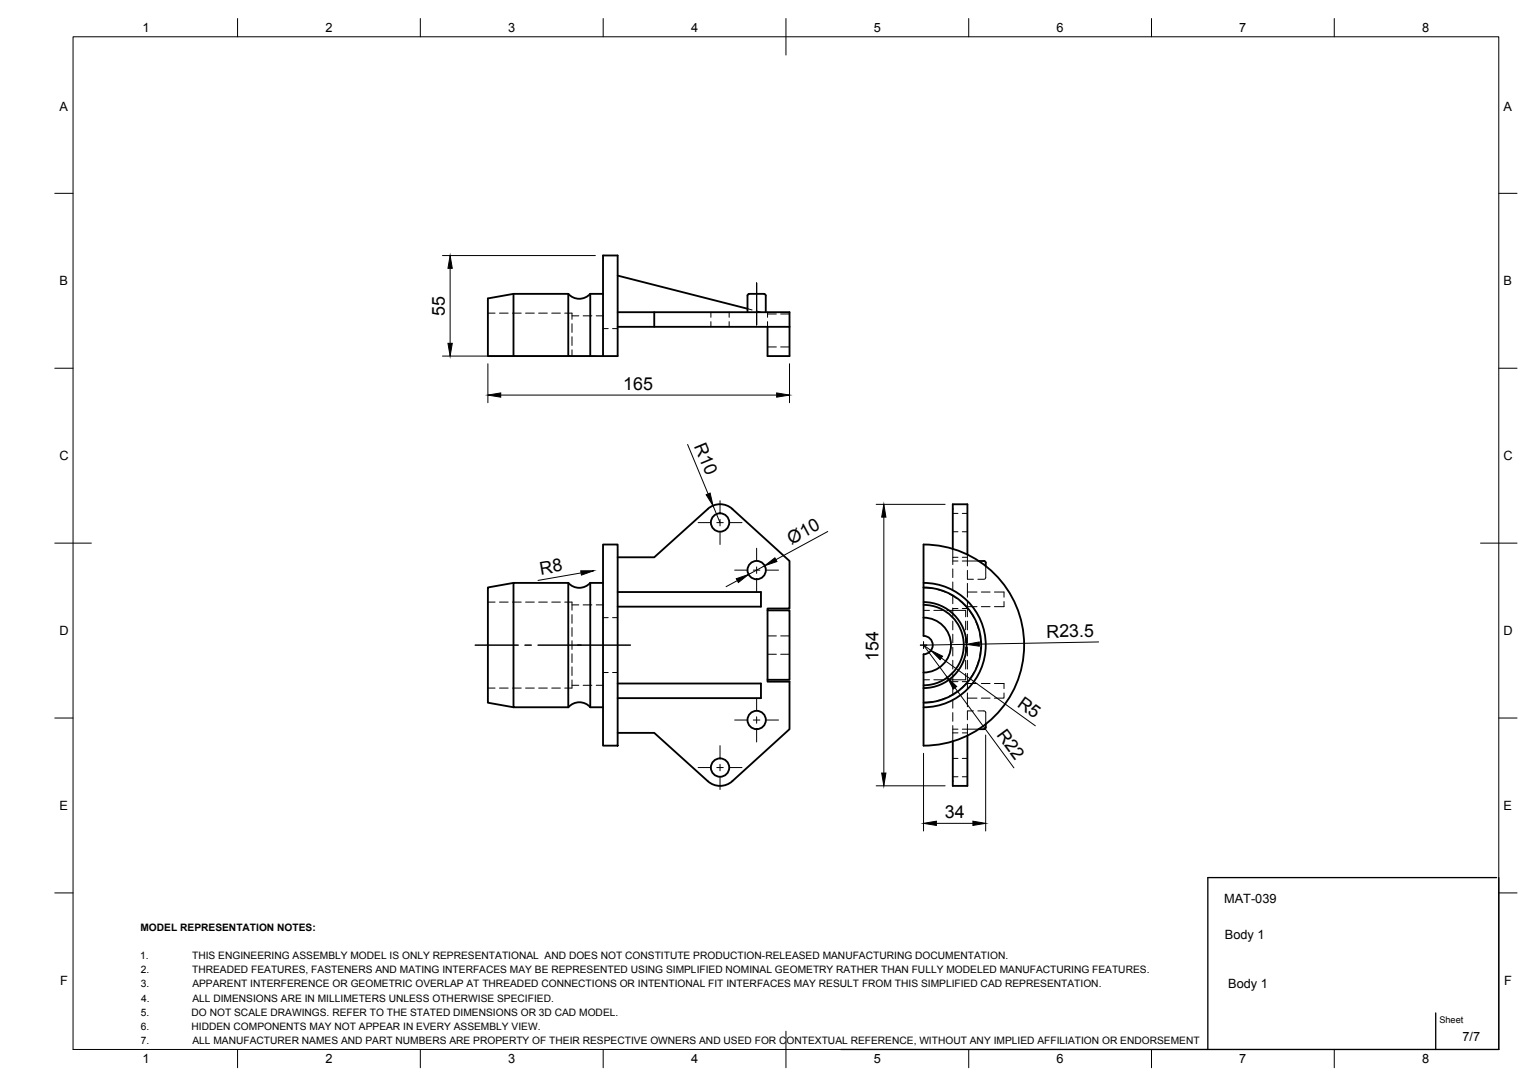
ISO-10303-21;
HEADER;
/* Generated by software containing ST-Developer
 * from STEP Tools, Inc. (www.steptools.com) 
 */

FILE_DESCRIPTION(
/* description */ ('STEP AP214'),
/* implementation_level */ '2;1');

FILE_NAME(
/* name */ 'Body 1.step',
/* time_stamp */ '2026-11-14T21:46:24-08:00',
/* author */ (''),
/* organization */ (''),
/* preprocessor_version */ 'ST-DEVELOPER v20.2',
/* originating_system */ 'Autodesk Translation Framework v15.17.0.0',
/* authorisation */ '');

FILE_SCHEMA (('AUTOMOTIVE_DESIGN { 1 0 10303 214 3 1 1 }'));
ENDSEC;

DATA;
#10=MECHANICAL_DESIGN_GEOMETRIC_PRESENTATION_REPRESENTATION('',(#89),#7783);
#75=SHAPE_REPRESENTATION_RELATIONSHIP('SRR','None',#7820,#82);
#82=ADVANCED_BREP_SHAPE_REPRESENTATION('',(#96),#7776);
#89=STYLED_ITEM('',(#7868),#96);
#96=MANIFOLD_SOLID_BREP('Body1',#4164);
#103=CONICAL_SURFACE('',#4303,34.,0.176708856070037);
#112=FACE_BOUND('',#1344,.T.);
#113=FACE_BOUND('',#1345,.T.);
#114=FACE_BOUND('',#1346,.T.);
#115=FACE_BOUND('',#1347,.T.);
#116=FACE_BOUND('',#1352,.T.);
#117=FACE_BOUND('',#1359,.T.);
#118=FACE_BOUND('',#1360,.T.);
#159=PLANE('',#4294);
#160=PLANE('',#4297);
#161=PLANE('',#4298);
#162=PLANE('',#4299);
#163=PLANE('',#4300);
#164=PLANE('',#4301);
#165=PLANE('',#4304);
#166=PLANE('',#4305);
#167=PLANE('',#4306);
#168=PLANE('',#4307);
#169=PLANE('',#4310);
#170=PLANE('',#4311);
#171=PLANE('',#4313);
#172=PLANE('',#4314);
#173=PLANE('',#4315);
#174=PLANE('',#4317);
#175=PLANE('',#4318);
#176=PLANE('',#4319);
#177=PLANE('',#4320);
#178=PLANE('',#4321);
#179=PLANE('',#4322);
#180=PLANE('',#4323);
#181=PLANE('',#4324);
#182=PLANE('',#4325);
#183=PLANE('',#4326);
#184=PLANE('',#4327);
#185=PLANE('',#4328);
#186=PLANE('',#4329);
#187=PLANE('',#4330);
#188=PLANE('',#4331);
#189=PLANE('',#4332);
#190=PLANE('',#4333);
#191=PLANE('',#4334);
#192=PLANE('',#4335);
#193=PLANE('',#4336);
#289=LINE('',#6018,#648);
#290=LINE('',#6028,#649);
#291=LINE('',#6034,#650);
#292=LINE('',#6037,#651);
#293=LINE('',#6042,#652);
#294=LINE('',#6048,#653);
#295=LINE('',#6055,#654);
#296=LINE('',#6058,#655);
#297=LINE('',#6064,#656);
#298=LINE('',#6067,#657);
#299=LINE('',#6073,#658);
#300=LINE('',#6076,#659);
#301=LINE('',#6082,#660);
#302=LINE('',#6085,#661);
#303=LINE('',#6090,#662);
#304=LINE('',#6091,#663);
#305=LINE('',#6094,#664);
#306=LINE('',#6097,#665);
#307=LINE('',#6101,#666);
#308=LINE('',#6103,#667);
#309=LINE('',#6105,#668);
#310=LINE('',#6107,#669);
#311=LINE('',#6109,#670);
#312=LINE('',#6113,#671);
#313=LINE('',#6115,#672);
#314=LINE('',#6117,#673);
#315=LINE('',#6119,#674);
#316=LINE('',#6121,#675);
#317=LINE('',#6123,#676);
#318=LINE('',#6125,#677);
#319=LINE('',#6127,#678);
#320=LINE('',#6129,#679);
#321=LINE('',#6131,#680);
#322=LINE('',#6133,#681);
#323=LINE('',#6135,#682);
#324=LINE('',#6137,#683);
#325=LINE('',#6141,#684);
#326=LINE('',#6142,#685);
#327=LINE('',#6145,#686);
#328=LINE('',#6146,#687);
#329=LINE('',#6147,#688);
#330=LINE('',#6148,#689);
#331=LINE('',#6149,#690);
#332=LINE('',#6150,#691);
#333=LINE('',#6154,#692);
#334=LINE('',#6156,#693);
#335=LINE('',#6158,#694);
#336=LINE('',#6160,#695);
#337=LINE('',#6162,#696);
#338=LINE('',#6163,#697);
#339=LINE('',#6164,#698);
#340=LINE('',#6168,#699);
#341=LINE('',#6169,#700);
#342=LINE('',#6170,#701);
#343=LINE('',#6172,#702);
#344=LINE('',#6174,#703);
#345=LINE('',#6176,#704);
#346=LINE('',#6177,#705);
#347=LINE('',#6179,#706);
#348=LINE('',#6181,#707);
#349=LINE('',#6182,#708);
#350=LINE('',#6184,#709);
#351=LINE('',#6186,#710);
#352=LINE('',#6187,#711);
#353=LINE('',#6191,#712);
#354=LINE('',#6193,#713);
#355=LINE('',#6195,#714);
#356=LINE('',#6197,#715);
#357=LINE('',#6199,#716);
#358=LINE('',#6201,#717);
#359=LINE('',#6203,#718);
#360=LINE('',#6207,#719);
#361=LINE('',#6208,#720);
#362=LINE('',#6210,#721);
#363=LINE('',#6212,#722);
#364=LINE('',#6216,#723);
#365=LINE('',#6218,#724);
#366=LINE('',#6219,#725);
#367=LINE('',#6220,#726);
#368=LINE('',#6222,#727);
#369=LINE('',#6224,#728);
#370=LINE('',#6226,#729);
#371=LINE('',#6229,#730);
#372=LINE('',#6230,#731);
#373=LINE('',#6232,#732);
#374=LINE('',#6234,#733);
#375=LINE('',#6236,#734);
#376=LINE('',#6239,#735);
#377=LINE('',#6240,#736);
#378=LINE('',#6244,#737);
#379=LINE('',#6245,#738);
#380=LINE('',#6252,#739);
#381=LINE('',#6253,#740);
#382=LINE('',#6255,#741);
#383=LINE('',#6256,#742);
#384=LINE('',#6259,#743);
#385=LINE('',#6261,#744);
#386=LINE('',#6263,#745);
#387=LINE('',#6265,#746);
#388=LINE('',#6266,#747);
#389=LINE('',#6268,#748);
#390=LINE('',#6269,#749);
#391=LINE('',#6271,#750);
#392=LINE('',#6273,#751);
#648=VECTOR('',#4740,5.00000000000003);
#649=VECTOR('',#4753,5.00000000000003);
#650=VECTOR('',#4758,1000.);
#651=VECTOR('',#4761,1000.);
#652=VECTOR('',#4766,5.00000000000002);
#653=VECTOR('',#4773,5.00000000000002);
#654=VECTOR('',#4780,1000.);
#655=VECTOR('',#4783,1000.);
#656=VECTOR('',#4788,1000.);
#657=VECTOR('',#4791,1000.);
#658=VECTOR('',#4796,1000.);
#659=VECTOR('',#4799,1000.);
#660=VECTOR('',#4804,1000.);
#661=VECTOR('',#4807,1000.);
#662=VECTOR('',#4812,1000.);
#663=VECTOR('',#4813,1000.);
#664=VECTOR('',#4816,1000.);
#665=VECTOR('',#4819,1000.);
#666=VECTOR('',#4822,1000.);
#667=VECTOR('',#4823,1000.);
#668=VECTOR('',#4824,1000.);
#669=VECTOR('',#4825,1000.);
#670=VECTOR('',#4826,1000.);
#671=VECTOR('',#4829,1000.);
#672=VECTOR('',#4830,1000.);
#673=VECTOR('',#4831,1000.);
#674=VECTOR('',#4832,1000.);
#675=VECTOR('',#4833,1000.);
#676=VECTOR('',#4834,1000.);
#677=VECTOR('',#4835,1000.);
#678=VECTOR('',#4836,1000.);
#679=VECTOR('',#4837,1000.);
#680=VECTOR('',#4838,1000.);
#681=VECTOR('',#4839,1000.);
#682=VECTOR('',#4840,1000.);
#683=VECTOR('',#4841,1000.);
#684=VECTOR('',#4844,1000.);
#685=VECTOR('',#4845,1000.);
#686=VECTOR('',#4848,1000.);
#687=VECTOR('',#4849,1000.);
#688=VECTOR('',#4850,1000.);
#689=VECTOR('',#4851,1000.);
#690=VECTOR('',#4852,1000.);
#691=VECTOR('',#4853,1000.);
#692=VECTOR('',#4856,1000.);
#693=VECTOR('',#4857,1000.);
#694=VECTOR('',#4858,1000.);
#695=VECTOR('',#4859,1000.);
#696=VECTOR('',#4860,1000.);
#697=VECTOR('',#4861,1000.);
#698=VECTOR('',#4862,1000.);
#699=VECTOR('',#4865,1000.);
#700=VECTOR('',#4866,1000.);
#701=VECTOR('',#4867,1000.);
#702=VECTOR('',#4870,1000.);
#703=VECTOR('',#4871,1000.);
#704=VECTOR('',#4872,1000.);
#705=VECTOR('',#4873,1000.);
#706=VECTOR('',#4874,1000.);
#707=VECTOR('',#4875,1000.);
#708=VECTOR('',#4876,1000.);
#709=VECTOR('',#4877,1000.);
#710=VECTOR('',#4878,1000.);
#711=VECTOR('',#4879,1000.);
#712=VECTOR('',#4884,1000.);
#713=VECTOR('',#4887,1000.);
#714=VECTOR('',#4890,1000.);
#715=VECTOR('',#4893,1000.);
#716=VECTOR('',#4896,1000.);
#717=VECTOR('',#4899,1000.);
#718=VECTOR('',#4900,1000.);
#719=VECTOR('',#4903,1000.);
#720=VECTOR('',#4904,1000.);
#721=VECTOR('',#4905,1000.);
#722=VECTOR('',#4906,1000.);
#723=VECTOR('',#4909,1000.);
#724=VECTOR('',#4910,1000.);
#725=VECTOR('',#4911,1000.);
#726=VECTOR('',#4912,1000.);
#727=VECTOR('',#4915,1000.);
#728=VECTOR('',#4918,1000.);
#729=VECTOR('',#4921,1000.);
#730=VECTOR('',#4926,1000.);
#731=VECTOR('',#4927,1000.);
#732=VECTOR('',#4930,1000.);
#733=VECTOR('',#4933,1000.);
#734=VECTOR('',#4936,1000.);
#735=VECTOR('',#4941,1000.);
#736=VECTOR('',#4942,1000.);
#737=VECTOR('',#4949,1000.);
#738=VECTOR('',#4950,1000.);
#739=VECTOR('',#4961,1000.);
#740=VECTOR('',#4962,1000.);
#741=VECTOR('',#4963,1000.);
#742=VECTOR('',#4964,1000.);
#743=VECTOR('',#4967,1000.);
#744=VECTOR('',#4968,1000.);
#745=VECTOR('',#4969,1000.);
#746=VECTOR('',#4970,1000.);
#747=VECTOR('',#4971,1000.);
#748=VECTOR('',#4974,1000.);
#749=VECTOR('',#4975,1000.);
#750=VECTOR('',#4978,1000.);
#751=VECTOR('',#4981,1000.);
#1007=CYLINDRICAL_SURFACE('',#4261,5.00000000000003);
#1008=CYLINDRICAL_SURFACE('',#4267,5.00000000000003);
#1009=CYLINDRICAL_SURFACE('',#4269,5.);
#1010=CYLINDRICAL_SURFACE('',#4272,5.00000000000002);
#1011=CYLINDRICAL_SURFACE('',#4275,5.00000000000002);
#1012=CYLINDRICAL_SURFACE('',#4278,23.5);
#1013=CYLINDRICAL_SURFACE('',#4281,22.);
#1014=CYLINDRICAL_SURFACE('',#4284,15.);
#1015=CYLINDRICAL_SURFACE('',#4287,55.);
#1016=CYLINDRICAL_SURFACE('',#4290,34.);
#1017=CYLINDRICAL_SURFACE('',#4292,34.);
#1018=CYLINDRICAL_SURFACE('',#4312,10.);
#1019=CYLINDRICAL_SURFACE('',#4316,10.);
#1086=FACE_OUTER_BOUND('',#1329,.T.);
#1087=FACE_OUTER_BOUND('',#1330,.T.);
#1088=FACE_OUTER_BOUND('',#1331,.T.);
#1089=FACE_OUTER_BOUND('',#1332,.T.);
#1090=FACE_OUTER_BOUND('',#1333,.T.);
#1091=FACE_OUTER_BOUND('',#1334,.T.);
#1092=FACE_OUTER_BOUND('',#1335,.T.);
#1093=FACE_OUTER_BOUND('',#1336,.T.);
#1094=FACE_OUTER_BOUND('',#1337,.T.);
#1095=FACE_OUTER_BOUND('',#1338,.T.);
#1096=FACE_OUTER_BOUND('',#1339,.T.);
#1097=FACE_OUTER_BOUND('',#1340,.T.);
#1098=FACE_OUTER_BOUND('',#1341,.T.);
#1099=FACE_OUTER_BOUND('',#1342,.T.);
#1100=FACE_OUTER_BOUND('',#1343,.T.);
#1101=FACE_OUTER_BOUND('',#1348,.T.);
#1102=FACE_OUTER_BOUND('',#1349,.T.);
#1103=FACE_OUTER_BOUND('',#1350,.T.);
#1104=FACE_OUTER_BOUND('',#1351,.T.);
#1105=FACE_OUTER_BOUND('',#1353,.T.);
#1106=FACE_OUTER_BOUND('',#1354,.T.);
#1107=FACE_OUTER_BOUND('',#1355,.T.);
#1108=FACE_OUTER_BOUND('',#1356,.T.);
#1109=FACE_OUTER_BOUND('',#1357,.T.);
#1110=FACE_OUTER_BOUND('',#1358,.T.);
#1111=FACE_OUTER_BOUND('',#1361,.T.);
#1112=FACE_OUTER_BOUND('',#1362,.T.);
#1113=FACE_OUTER_BOUND('',#1363,.T.);
#1114=FACE_OUTER_BOUND('',#1364,.T.);
#1115=FACE_OUTER_BOUND('',#1365,.T.);
#1116=FACE_OUTER_BOUND('',#1366,.T.);
#1117=FACE_OUTER_BOUND('',#1367,.T.);
#1118=FACE_OUTER_BOUND('',#1368,.T.);
#1119=FACE_OUTER_BOUND('',#1369,.T.);
#1120=FACE_OUTER_BOUND('',#1370,.T.);
#1121=FACE_OUTER_BOUND('',#1371,.T.);
#1122=FACE_OUTER_BOUND('',#1372,.T.);
#1123=FACE_OUTER_BOUND('',#1373,.T.);
#1124=FACE_OUTER_BOUND('',#1374,.T.);
#1125=FACE_OUTER_BOUND('',#1375,.T.);
#1126=FACE_OUTER_BOUND('',#1376,.T.);
#1127=FACE_OUTER_BOUND('',#1377,.T.);
#1128=FACE_OUTER_BOUND('',#1378,.T.);
#1129=FACE_OUTER_BOUND('',#1379,.T.);
#1130=FACE_OUTER_BOUND('',#1380,.T.);
#1131=FACE_OUTER_BOUND('',#1381,.T.);
#1132=FACE_OUTER_BOUND('',#1382,.T.);
#1133=FACE_OUTER_BOUND('',#1383,.T.);
#1134=FACE_OUTER_BOUND('',#1384,.T.);
#1135=FACE_OUTER_BOUND('',#1385,.T.);
#1136=FACE_OUTER_BOUND('',#1386,.T.);
#1137=FACE_OUTER_BOUND('',#1387,.T.);
#1329=EDGE_LOOP('',(#2758,#2759,#2760,#2761));
#1330=EDGE_LOOP('',(#2762,#2763,#2764,#2765));
#1331=EDGE_LOOP('',(#2766,#2767,#2768,#2769));
#1332=EDGE_LOOP('',(#2770,#2771,#2772,#2773));
#1333=EDGE_LOOP('',(#2774,#2775,#2776,#2777));
#1334=EDGE_LOOP('',(#2778,#2779,#2780,#2781));
#1335=EDGE_LOOP('',(#2782,#2783,#2784,#2785));
#1336=EDGE_LOOP('',(#2786,#2787,#2788,#2789));
#1337=EDGE_LOOP('',(#2790,#2791,#2792,#2793));
#1338=EDGE_LOOP('',(#2794,#2795,#2796,#2797));
#1339=EDGE_LOOP('',(#2798,#2799,#2800,#2801));
#1340=EDGE_LOOP('',(#2802,#2803,#2804,#2805));
#1341=EDGE_LOOP('',(#2806,#2807,#2808,#2809));
#1342=EDGE_LOOP('',(#2810,#2811,#2812,#2813));
#1343=EDGE_LOOP('',(#2814,#2815,#2816,#2817,#2818,#2819,#2820,#2821,#2822,
#2823,#2824,#2825,#2826,#2827,#2828,#2829,#2830,#2831,#2832,#2833,#2834,
#2835));
#1344=EDGE_LOOP('',(#2836));
#1345=EDGE_LOOP('',(#2837));
#1346=EDGE_LOOP('',(#2838));
#1347=EDGE_LOOP('',(#2839));
#1348=EDGE_LOOP('',(#2840,#2841,#2842,#2843,#2844,#2845,#2846,#2847,#2848,
#2849,#2850,#2851,#2852));
#1349=EDGE_LOOP('',(#2853,#2854,#2855,#2856,#2857,#2858,#2859,#2860));
#1350=EDGE_LOOP('',(#2861,#2862,#2863,#2864));
#1351=EDGE_LOOP('',(#2865,#2866,#2867,#2868));
#1352=EDGE_LOOP('',(#2869,#2870,#2871,#2872,#2873,#2874,#2875,#2876,#2877,
#2878,#2879,#2880));
#1353=EDGE_LOOP('',(#2881,#2882,#2883,#2884));
#1354=EDGE_LOOP('',(#2885,#2886,#2887,#2888));
#1355=EDGE_LOOP('',(#2889,#2890,#2891,#2892));
#1356=EDGE_LOOP('',(#2893,#2894,#2895,#2896));
#1357=EDGE_LOOP('',(#2897,#2898,#2899,#2900));
#1358=EDGE_LOOP('',(#2901,#2902,#2903,#2904,#2905,#2906,#2907,#2908,#2909,
#2910,#2911,#2912,#2913,#2914,#2915,#2916));
#1359=EDGE_LOOP('',(#2917));
#1360=EDGE_LOOP('',(#2918));
#1361=EDGE_LOOP('',(#2919,#2920,#2921,#2922));
#1362=EDGE_LOOP('',(#2923,#2924,#2925,#2926));
#1363=EDGE_LOOP('',(#2927,#2928,#2929,#2930));
#1364=EDGE_LOOP('',(#2931,#2932,#2933,#2934));
#1365=EDGE_LOOP('',(#2935,#2936,#2937,#2938));
#1366=EDGE_LOOP('',(#2939,#2940,#2941,#2942));
#1367=EDGE_LOOP('',(#2943,#2944,#2945,#2946));
#1368=EDGE_LOOP('',(#2947,#2948,#2949,#2950));
#1369=EDGE_LOOP('',(#2951,#2952,#2953,#2954));
#1370=EDGE_LOOP('',(#2955,#2956,#2957,#2958));
#1371=EDGE_LOOP('',(#2959,#2960,#2961));
#1372=EDGE_LOOP('',(#2962,#2963,#2964));
#1373=EDGE_LOOP('',(#2965,#2966,#2967,#2968));
#1374=EDGE_LOOP('',(#2969,#2970,#2971));
#1375=EDGE_LOOP('',(#2972,#2973,#2974));
#1376=EDGE_LOOP('',(#2975,#2976,#2977,#2978));
#1377=EDGE_LOOP('',(#2979,#2980,#2981,#2982));
#1378=EDGE_LOOP('',(#2983,#2984,#2985,#2986,#2987,#2988));
#1379=EDGE_LOOP('',(#2989,#2990,#2991,#2992,#2993,#2994));
#1380=EDGE_LOOP('',(#2995,#2996,#2997,#2998));
#1381=EDGE_LOOP('',(#2999,#3000,#3001,#3002,#3003));
#1382=EDGE_LOOP('',(#3004,#3005,#3006,#3007,#3008));
#1383=EDGE_LOOP('',(#3009,#3010,#3011,#3012));
#1384=EDGE_LOOP('',(#3013,#3014,#3015,#3016,#3017,#3018,#3019,#3020,#3021,
#3022,#3023,#3024,#3025));
#1385=EDGE_LOOP('',(#3026,#3027,#3028,#3029));
#1386=EDGE_LOOP('',(#3030));
#1387=EDGE_LOOP('',(#3031));
#1619=CIRCLE('',#4253,8.);
#1620=CIRCLE('',#4254,34.);
#1621=CIRCLE('',#4255,8.);
#1622=CIRCLE('',#4256,34.);
#1623=CIRCLE('',#4258,5.00000000000003);
#1624=CIRCLE('',#4259,1.);
#1625=CIRCLE('',#4260,4.00000000000003);
#1626=CIRCLE('',#4262,5.00000000000003);
#1627=CIRCLE('',#4264,5.00000000000003);
#1628=CIRCLE('',#4265,1.);
#1629=CIRCLE('',#4266,4.00000000000003);
#1630=CIRCLE('',#4268,5.00000000000003);
#1631=CIRCLE('',#4270,5.);
#1632=CIRCLE('',#4271,5.);
#1633=CIRCLE('',#4273,5.00000000000002);
#1634=CIRCLE('',#4274,5.00000000000002);
#1635=CIRCLE('',#4276,5.00000000000003);
#1636=CIRCLE('',#4277,5.00000000000003);
#1637=CIRCLE('',#4279,23.5);
#1638=CIRCLE('',#4280,23.5);
#1639=CIRCLE('',#4282,22.);
#1640=CIRCLE('',#4283,22.);
#1641=CIRCLE('',#4285,15.);
#1642=CIRCLE('',#4286,15.);
#1643=CIRCLE('',#4288,55.);
#1644=CIRCLE('',#4289,55.);
#1645=CIRCLE('',#4291,34.);
#1646=CIRCLE('',#4293,34.);
#1647=CIRCLE('',#4295,10.);
#1648=CIRCLE('',#4296,10.);
#1649=CIRCLE('',#4302,31.5);
#1650=CIRCLE('',#4308,10.);
#1651=CIRCLE('',#4309,10.);
#1822=VERTEX_POINT('',#6001);
#1823=VERTEX_POINT('',#6002);
#1824=VERTEX_POINT('',#6004);
#1825=VERTEX_POINT('',#6006);
#1826=VERTEX_POINT('',#6010);
#1827=VERTEX_POINT('',#6012);
#1828=VERTEX_POINT('',#6016);
#1829=VERTEX_POINT('',#6020);
#1830=VERTEX_POINT('',#6022);
#1831=VERTEX_POINT('',#6026);
#1832=VERTEX_POINT('',#6030);
#1833=VERTEX_POINT('',#6031);
#1834=VERTEX_POINT('',#6033);
#1835=VERTEX_POINT('',#6035);
#1836=VERTEX_POINT('',#6039);
#1837=VERTEX_POINT('',#6041);
#1838=VERTEX_POINT('',#6045);
#1839=VERTEX_POINT('',#6047);
#1840=VERTEX_POINT('',#6051);
#1841=VERTEX_POINT('',#6052);
#1842=VERTEX_POINT('',#6054);
#1843=VERTEX_POINT('',#6056);
#1844=VERTEX_POINT('',#6060);
#1845=VERTEX_POINT('',#6061);
#1846=VERTEX_POINT('',#6063);
#1847=VERTEX_POINT('',#6065);
#1848=VERTEX_POINT('',#6069);
#1849=VERTEX_POINT('',#6070);
#1850=VERTEX_POINT('',#6072);
#1851=VERTEX_POINT('',#6074);
#1852=VERTEX_POINT('',#6078);
#1853=VERTEX_POINT('',#6079);
#1854=VERTEX_POINT('',#6081);
#1855=VERTEX_POINT('',#6083);
#1856=VERTEX_POINT('',#6087);
#1857=VERTEX_POINT('',#6088);
#1858=VERTEX_POINT('',#6093);
#1859=VERTEX_POINT('',#6095);
#1860=VERTEX_POINT('',#6099);
#1861=VERTEX_POINT('',#6100);
#1862=VERTEX_POINT('',#6102);
#1863=VERTEX_POINT('',#6104);
#1864=VERTEX_POINT('',#6106);
#1865=VERTEX_POINT('',#6108);
#1866=VERTEX_POINT('',#6110);
#1867=VERTEX_POINT('',#6112);
#1868=VERTEX_POINT('',#6114);
#1869=VERTEX_POINT('',#6116);
#1870=VERTEX_POINT('',#6118);
#1871=VERTEX_POINT('',#6120);
#1872=VERTEX_POINT('',#6122);
#1873=VERTEX_POINT('',#6124);
#1874=VERTEX_POINT('',#6126);
#1875=VERTEX_POINT('',#6128);
#1876=VERTEX_POINT('',#6130);
#1877=VERTEX_POINT('',#6132);
#1878=VERTEX_POINT('',#6134);
#1879=VERTEX_POINT('',#6136);
#1880=VERTEX_POINT('',#6138);
#1881=VERTEX_POINT('',#6140);
#1882=VERTEX_POINT('',#6144);
#1883=VERTEX_POINT('',#6152);
#1884=VERTEX_POINT('',#6153);
#1885=VERTEX_POINT('',#6155);
#1886=VERTEX_POINT('',#6157);
#1887=VERTEX_POINT('',#6159);
#1888=VERTEX_POINT('',#6161);
#1889=VERTEX_POINT('',#6166);
#1890=VERTEX_POINT('',#6167);
#1891=VERTEX_POINT('',#6173);
#1892=VERTEX_POINT('',#6175);
#1893=VERTEX_POINT('',#6178);
#1894=VERTEX_POINT('',#6180);
#1895=VERTEX_POINT('',#6183);
#1896=VERTEX_POINT('',#6185);
#1897=VERTEX_POINT('',#6189);
#1898=VERTEX_POINT('',#6202);
#1899=VERTEX_POINT('',#6204);
#1900=VERTEX_POINT('',#6206);
#1901=VERTEX_POINT('',#6209);
#1902=VERTEX_POINT('',#6211);
#1903=VERTEX_POINT('',#6213);
#1904=VERTEX_POINT('',#6215);
#1905=VERTEX_POINT('',#6217);
#1906=VERTEX_POINT('',#6251);
#1907=VERTEX_POINT('',#6254);
#1908=VERTEX_POINT('',#6258);
#1909=VERTEX_POINT('',#6260);
#1910=VERTEX_POINT('',#6262);
#1911=VERTEX_POINT('',#6264);
#2186=EDGE_CURVE('',#1822,#1823,#1619,.T.);
#2187=EDGE_CURVE('',#1823,#1824,#1620,.T.);
#2188=EDGE_CURVE('',#1824,#1825,#1621,.T.);
#2189=EDGE_CURVE('',#1822,#1825,#1622,.T.);
#2190=EDGE_CURVE('',#1826,#1826,#1623,.T.);
#2191=EDGE_CURVE('',#1826,#1827,#1624,.T.);
#2192=EDGE_CURVE('',#1827,#1827,#1625,.T.);
#2193=EDGE_CURVE('',#1828,#1828,#1626,.T.);
#2194=EDGE_CURVE('',#1828,#1826,#289,.T.);
#2195=EDGE_CURVE('',#1829,#1829,#1627,.T.);
#2196=EDGE_CURVE('',#1829,#1830,#1628,.T.);
#2197=EDGE_CURVE('',#1830,#1830,#1629,.T.);
#2198=EDGE_CURVE('',#1831,#1831,#1630,.T.);
#2199=EDGE_CURVE('',#1831,#1829,#290,.T.);
#2200=EDGE_CURVE('',#1832,#1833,#1631,.T.);
#2201=EDGE_CURVE('',#1834,#1833,#291,.T.);
#2202=EDGE_CURVE('',#1835,#1834,#1632,.T.);
#2203=EDGE_CURVE('',#1832,#1835,#292,.T.);
#2204=EDGE_CURVE('',#1836,#1836,#1633,.T.);
#2205=EDGE_CURVE('',#1836,#1837,#293,.T.);
#2206=EDGE_CURVE('',#1837,#1837,#1634,.T.);
#2207=EDGE_CURVE('',#1838,#1838,#1635,.T.);
#2208=EDGE_CURVE('',#1838,#1839,#294,.T.);
#2209=EDGE_CURVE('',#1839,#1839,#1636,.T.);
#2210=EDGE_CURVE('',#1840,#1841,#1637,.T.);
#2211=EDGE_CURVE('',#1840,#1842,#295,.T.);
#2212=EDGE_CURVE('',#1842,#1843,#1638,.T.);
#2213=EDGE_CURVE('',#1843,#1841,#296,.T.);
#2214=EDGE_CURVE('',#1844,#1845,#1639,.T.);
#2215=EDGE_CURVE('',#1844,#1846,#297,.T.);
#2216=EDGE_CURVE('',#1846,#1847,#1640,.T.);
#2217=EDGE_CURVE('',#1847,#1845,#298,.T.);
#2218=EDGE_CURVE('',#1848,#1849,#1641,.T.);
#2219=EDGE_CURVE('',#1848,#1850,#299,.T.);
#2220=EDGE_CURVE('',#1850,#1851,#1642,.T.);
#2221=EDGE_CURVE('',#1851,#1849,#300,.T.);
#2222=EDGE_CURVE('',#1852,#1853,#1643,.T.);
#2223=EDGE_CURVE('',#1853,#1854,#301,.T.);
#2224=EDGE_CURVE('',#1855,#1854,#1644,.T.);
#2225=EDGE_CURVE('',#1855,#1852,#302,.T.);
#2226=EDGE_CURVE('',#1856,#1857,#1645,.T.);
#2227=EDGE_CURVE('',#1857,#1824,#303,.T.);
#2228=EDGE_CURVE('',#1823,#1856,#304,.T.);
#2229=EDGE_CURVE('',#1825,#1858,#305,.T.);
#2230=EDGE_CURVE('',#1859,#1858,#1646,.T.);
#2231=EDGE_CURVE('',#1859,#1822,#306,.T.);
#2232=EDGE_CURVE('',#1860,#1861,#307,.T.);
#2233=EDGE_CURVE('',#1862,#1860,#308,.T.);
#2234=EDGE_CURVE('',#1862,#1863,#309,.T.);
#2235=EDGE_CURVE('',#1863,#1864,#310,.T.);
#2236=EDGE_CURVE('',#1864,#1865,#311,.T.);
#2237=EDGE_CURVE('',#1865,#1866,#1647,.T.);
#2238=EDGE_CURVE('',#1866,#1867,#312,.T.);
#2239=EDGE_CURVE('',#1867,#1868,#313,.T.);
#2240=EDGE_CURVE('',#1868,#1869,#314,.T.);
#2241=EDGE_CURVE('',#1870,#1869,#315,.T.);
#2242=EDGE_CURVE('',#1870,#1871,#316,.T.);
#2243=EDGE_CURVE('',#1871,#1872,#317,.T.);
#2244=EDGE_CURVE('',#1872,#1873,#318,.T.);
#2245=EDGE_CURVE('',#1874,#1873,#319,.T.);
#2246=EDGE_CURVE('',#1875,#1874,#320,.T.);
#2247=EDGE_CURVE('',#1875,#1876,#321,.T.);
#2248=EDGE_CURVE('',#1876,#1877,#322,.T.);
#2249=EDGE_CURVE('',#1877,#1878,#323,.T.);
#2250=EDGE_CURVE('',#1878,#1879,#324,.T.);
#2251=EDGE_CURVE('',#1879,#1880,#1648,.T.);
#2252=EDGE_CURVE('',#1880,#1881,#325,.T.);
#2253=EDGE_CURVE('',#1881,#1861,#326,.T.);
#2254=EDGE_CURVE('',#1858,#1882,#327,.T.);
#2255=EDGE_CURVE('',#1854,#1857,#328,.T.);
#2256=EDGE_CURVE('',#1849,#1853,#329,.T.);
#2257=EDGE_CURVE('',#1845,#1851,#330,.T.);
#2258=EDGE_CURVE('',#1841,#1847,#331,.T.);
#2259=EDGE_CURVE('',#1882,#1843,#332,.T.);
#2260=EDGE_CURVE('',#1883,#1884,#333,.T.);
#2261=EDGE_CURVE('',#1885,#1884,#334,.T.);
#2262=EDGE_CURVE('',#1886,#1885,#335,.T.);
#2263=EDGE_CURVE('',#1886,#1887,#336,.T.);
#2264=EDGE_CURVE('',#1887,#1888,#337,.T.);
#2265=EDGE_CURVE('',#1888,#1862,#338,.T.);
#2266=EDGE_CURVE('',#1860,#1883,#339,.T.);
#2267=EDGE_CURVE('',#1889,#1890,#340,.T.);
#2268=EDGE_CURVE('',#1861,#1890,#341,.T.);
#2269=EDGE_CURVE('',#1881,#1889,#342,.T.);
#2270=EDGE_CURVE('',#1852,#1848,#343,.T.);
#2271=EDGE_CURVE('',#1876,#1891,#344,.T.);
#2272=EDGE_CURVE('',#1891,#1892,#345,.T.);
#2273=EDGE_CURVE('',#1873,#1892,#346,.T.);
#2274=EDGE_CURVE('',#1872,#1893,#347,.T.);
#2275=EDGE_CURVE('',#1894,#1893,#348,.T.);
#2276=EDGE_CURVE('',#1869,#1894,#349,.T.);
#2277=EDGE_CURVE('',#1868,#1895,#350,.T.);
#2278=EDGE_CURVE('',#1895,#1896,#351,.T.);
#2279=EDGE_CURVE('',#1877,#1896,#352,.T.);
#2280=EDGE_CURVE('',#1897,#1882,#1649,.T.);
#2281=EDGE_CURVE('',#1842,#1897,#353,.T.);
#2282=EDGE_CURVE('',#1897,#1859,#354,.T.);
#2283=EDGE_CURVE('',#1856,#1855,#355,.T.);
#2284=EDGE_CURVE('',#1850,#1844,#356,.T.);
#2285=EDGE_CURVE('',#1846,#1840,#357,.T.);
#2286=EDGE_CURVE('',#1883,#1890,#358,.T.);
#2287=EDGE_CURVE('',#1898,#1889,#359,.T.);
#2288=EDGE_CURVE('',#1899,#1898,#1650,.T.);
#2289=EDGE_CURVE('',#1900,#1899,#360,.T.);
#2290=EDGE_CURVE('',#1896,#1900,#361,.T.);
#2291=EDGE_CURVE('',#1901,#1895,#362,.T.);
#2292=EDGE_CURVE('',#1902,#1901,#363,.T.);
#2293=EDGE_CURVE('',#1903,#1902,#1651,.T.);
#2294=EDGE_CURVE('',#1904,#1903,#364,.T.);
#2295=EDGE_CURVE('',#1905,#1904,#365,.T.);
#2296=EDGE_CURVE('',#1905,#1888,#366,.T.);
#2297=EDGE_CURVE('',#1884,#1887,#367,.T.);
#2298=EDGE_CURVE('',#1878,#1900,#368,.T.);
#2299=EDGE_CURVE('',#1879,#1899,#369,.T.);
#2300=EDGE_CURVE('',#1880,#1898,#370,.T.);
#2301=EDGE_CURVE('',#1905,#1863,#371,.T.);
#2302=EDGE_CURVE('',#1864,#1904,#372,.T.);
#2303=EDGE_CURVE('',#1865,#1903,#373,.T.);
#2304=EDGE_CURVE('',#1866,#1902,#374,.T.);
#2305=EDGE_CURVE('',#1867,#1901,#375,.T.);
#2306=EDGE_CURVE('',#1893,#1871,#376,.T.);
#2307=EDGE_CURVE('',#1894,#1870,#377,.T.);
#2308=EDGE_CURVE('',#1892,#1874,#378,.T.);
#2309=EDGE_CURVE('',#1891,#1875,#379,.T.);
#2310=EDGE_CURVE('',#1906,#1887,#380,.T.);
#2311=EDGE_CURVE('',#1906,#1835,#381,.T.);
#2312=EDGE_CURVE('',#1834,#1907,#382,.T.);
#2313=EDGE_CURVE('',#1884,#1907,#383,.T.);
#2314=EDGE_CURVE('',#1908,#1832,#384,.T.);
#2315=EDGE_CURVE('',#1908,#1909,#385,.T.);
#2316=EDGE_CURVE('',#1909,#1910,#386,.T.);
#2317=EDGE_CURVE('',#1910,#1911,#387,.T.);
#2318=EDGE_CURVE('',#1833,#1911,#388,.T.);
#2319=EDGE_CURVE('',#1910,#1885,#389,.T.);
#2320=EDGE_CURVE('',#1909,#1886,#390,.T.);
#2321=EDGE_CURVE('',#1907,#1911,#391,.T.);
#2322=EDGE_CURVE('',#1908,#1906,#392,.T.);
#2758=ORIENTED_EDGE('',*,*,#2186,.T.);
#2759=ORIENTED_EDGE('',*,*,#2187,.T.);
#2760=ORIENTED_EDGE('',*,*,#2188,.T.);
#2761=ORIENTED_EDGE('',*,*,#2189,.F.);
#2762=ORIENTED_EDGE('',*,*,#2190,.F.);
#2763=ORIENTED_EDGE('',*,*,#2191,.T.);
#2764=ORIENTED_EDGE('',*,*,#2192,.F.);
#2765=ORIENTED_EDGE('',*,*,#2191,.F.);
#2766=ORIENTED_EDGE('',*,*,#2193,.F.);
#2767=ORIENTED_EDGE('',*,*,#2194,.T.);
#2768=ORIENTED_EDGE('',*,*,#2190,.T.);
#2769=ORIENTED_EDGE('',*,*,#2194,.F.);
#2770=ORIENTED_EDGE('',*,*,#2195,.F.);
#2771=ORIENTED_EDGE('',*,*,#2196,.T.);
#2772=ORIENTED_EDGE('',*,*,#2197,.F.);
#2773=ORIENTED_EDGE('',*,*,#2196,.F.);
#2774=ORIENTED_EDGE('',*,*,#2198,.T.);
#2775=ORIENTED_EDGE('',*,*,#2199,.T.);
#2776=ORIENTED_EDGE('',*,*,#2195,.T.);
#2777=ORIENTED_EDGE('',*,*,#2199,.F.);
#2778=ORIENTED_EDGE('',*,*,#2200,.T.);
#2779=ORIENTED_EDGE('',*,*,#2201,.F.);
#2780=ORIENTED_EDGE('',*,*,#2202,.F.);
#2781=ORIENTED_EDGE('',*,*,#2203,.F.);
#2782=ORIENTED_EDGE('',*,*,#2204,.T.);
#2783=ORIENTED_EDGE('',*,*,#2205,.T.);
#2784=ORIENTED_EDGE('',*,*,#2206,.F.);
#2785=ORIENTED_EDGE('',*,*,#2205,.F.);
#2786=ORIENTED_EDGE('',*,*,#2207,.T.);
#2787=ORIENTED_EDGE('',*,*,#2208,.T.);
#2788=ORIENTED_EDGE('',*,*,#2209,.F.);
#2789=ORIENTED_EDGE('',*,*,#2208,.F.);
#2790=ORIENTED_EDGE('',*,*,#2210,.F.);
#2791=ORIENTED_EDGE('',*,*,#2211,.T.);
#2792=ORIENTED_EDGE('',*,*,#2212,.T.);
#2793=ORIENTED_EDGE('',*,*,#2213,.T.);
#2794=ORIENTED_EDGE('',*,*,#2214,.F.);
#2795=ORIENTED_EDGE('',*,*,#2215,.T.);
#2796=ORIENTED_EDGE('',*,*,#2216,.T.);
#2797=ORIENTED_EDGE('',*,*,#2217,.T.);
#2798=ORIENTED_EDGE('',*,*,#2218,.F.);
#2799=ORIENTED_EDGE('',*,*,#2219,.T.);
#2800=ORIENTED_EDGE('',*,*,#2220,.T.);
#2801=ORIENTED_EDGE('',*,*,#2221,.T.);
#2802=ORIENTED_EDGE('',*,*,#2222,.T.);
#2803=ORIENTED_EDGE('',*,*,#2223,.T.);
#2804=ORIENTED_EDGE('',*,*,#2224,.F.);
#2805=ORIENTED_EDGE('',*,*,#2225,.T.);
#2806=ORIENTED_EDGE('',*,*,#2226,.T.);
#2807=ORIENTED_EDGE('',*,*,#2227,.T.);
#2808=ORIENTED_EDGE('',*,*,#2187,.F.);
#2809=ORIENTED_EDGE('',*,*,#2228,.T.);
#2810=ORIENTED_EDGE('',*,*,#2189,.T.);
#2811=ORIENTED_EDGE('',*,*,#2229,.T.);
#2812=ORIENTED_EDGE('',*,*,#2230,.F.);
#2813=ORIENTED_EDGE('',*,*,#2231,.T.);
#2814=ORIENTED_EDGE('',*,*,#2232,.F.);
#2815=ORIENTED_EDGE('',*,*,#2233,.F.);
#2816=ORIENTED_EDGE('',*,*,#2234,.T.);
#2817=ORIENTED_EDGE('',*,*,#2235,.T.);
#2818=ORIENTED_EDGE('',*,*,#2236,.T.);
#2819=ORIENTED_EDGE('',*,*,#2237,.T.);
#2820=ORIENTED_EDGE('',*,*,#2238,.T.);
#2821=ORIENTED_EDGE('',*,*,#2239,.T.);
#2822=ORIENTED_EDGE('',*,*,#2240,.T.);
#2823=ORIENTED_EDGE('',*,*,#2241,.F.);
#2824=ORIENTED_EDGE('',*,*,#2242,.T.);
#2825=ORIENTED_EDGE('',*,*,#2243,.T.);
#2826=ORIENTED_EDGE('',*,*,#2244,.T.);
#2827=ORIENTED_EDGE('',*,*,#2245,.F.);
#2828=ORIENTED_EDGE('',*,*,#2246,.F.);
#2829=ORIENTED_EDGE('',*,*,#2247,.T.);
#2830=ORIENTED_EDGE('',*,*,#2248,.T.);
#2831=ORIENTED_EDGE('',*,*,#2249,.T.);
#2832=ORIENTED_EDGE('',*,*,#2250,.T.);
#2833=ORIENTED_EDGE('',*,*,#2251,.T.);
#2834=ORIENTED_EDGE('',*,*,#2252,.T.);
#2835=ORIENTED_EDGE('',*,*,#2253,.T.);
#2836=ORIENTED_EDGE('',*,*,#2193,.T.);
#2837=ORIENTED_EDGE('',*,*,#2198,.F.);
#2838=ORIENTED_EDGE('',*,*,#2207,.F.);
#2839=ORIENTED_EDGE('',*,*,#2204,.F.);
#2840=ORIENTED_EDGE('',*,*,#2254,.F.);
#2841=ORIENTED_EDGE('',*,*,#2229,.F.);
#2842=ORIENTED_EDGE('',*,*,#2188,.F.);
#2843=ORIENTED_EDGE('',*,*,#2227,.F.);
#2844=ORIENTED_EDGE('',*,*,#2255,.F.);
#2845=ORIENTED_EDGE('',*,*,#2223,.F.);
#2846=ORIENTED_EDGE('',*,*,#2256,.F.);
#2847=ORIENTED_EDGE('',*,*,#2221,.F.);
#2848=ORIENTED_EDGE('',*,*,#2257,.F.);
#2849=ORIENTED_EDGE('',*,*,#2217,.F.);
#2850=ORIENTED_EDGE('',*,*,#2258,.F.);
#2851=ORIENTED_EDGE('',*,*,#2213,.F.);
#2852=ORIENTED_EDGE('',*,*,#2259,.F.);
#2853=ORIENTED_EDGE('',*,*,#2260,.T.);
#2854=ORIENTED_EDGE('',*,*,#2261,.F.);
#2855=ORIENTED_EDGE('',*,*,#2262,.F.);
#2856=ORIENTED_EDGE('',*,*,#2263,.T.);
#2857=ORIENTED_EDGE('',*,*,#2264,.T.);
#2858=ORIENTED_EDGE('',*,*,#2265,.T.);
#2859=ORIENTED_EDGE('',*,*,#2233,.T.);
#2860=ORIENTED_EDGE('',*,*,#2266,.T.);
#2861=ORIENTED_EDGE('',*,*,#2267,.T.);
#2862=ORIENTED_EDGE('',*,*,#2268,.F.);
#2863=ORIENTED_EDGE('',*,*,#2253,.F.);
#2864=ORIENTED_EDGE('',*,*,#2269,.T.);
#2865=ORIENTED_EDGE('',*,*,#2222,.F.);
#2866=ORIENTED_EDGE('',*,*,#2270,.T.);
#2867=ORIENTED_EDGE('',*,*,#2218,.T.);
#2868=ORIENTED_EDGE('',*,*,#2256,.T.);
#2869=ORIENTED_EDGE('',*,*,#2271,.T.);
#2870=ORIENTED_EDGE('',*,*,#2272,.T.);
#2871=ORIENTED_EDGE('',*,*,#2273,.F.);
#2872=ORIENTED_EDGE('',*,*,#2244,.F.);
#2873=ORIENTED_EDGE('',*,*,#2274,.T.);
#2874=ORIENTED_EDGE('',*,*,#2275,.F.);
#2875=ORIENTED_EDGE('',*,*,#2276,.F.);
#2876=ORIENTED_EDGE('',*,*,#2240,.F.);
#2877=ORIENTED_EDGE('',*,*,#2277,.T.);
#2878=ORIENTED_EDGE('',*,*,#2278,.T.);
#2879=ORIENTED_EDGE('',*,*,#2279,.F.);
#2880=ORIENTED_EDGE('',*,*,#2248,.F.);
#2881=ORIENTED_EDGE('',*,*,#2280,.T.);
#2882=ORIENTED_EDGE('',*,*,#2259,.T.);
#2883=ORIENTED_EDGE('',*,*,#2212,.F.);
#2884=ORIENTED_EDGE('',*,*,#2281,.T.);
#2885=ORIENTED_EDGE('',*,*,#2280,.F.);
#2886=ORIENTED_EDGE('',*,*,#2282,.T.);
#2887=ORIENTED_EDGE('',*,*,#2230,.T.);
#2888=ORIENTED_EDGE('',*,*,#2254,.T.);
#2889=ORIENTED_EDGE('',*,*,#2224,.T.);
#2890=ORIENTED_EDGE('',*,*,#2255,.T.);
#2891=ORIENTED_EDGE('',*,*,#2226,.F.);
#2892=ORIENTED_EDGE('',*,*,#2283,.T.);
#2893=ORIENTED_EDGE('',*,*,#2214,.T.);
#2894=ORIENTED_EDGE('',*,*,#2257,.T.);
#2895=ORIENTED_EDGE('',*,*,#2220,.F.);
#2896=ORIENTED_EDGE('',*,*,#2284,.T.);
#2897=ORIENTED_EDGE('',*,*,#2210,.T.);
#2898=ORIENTED_EDGE('',*,*,#2258,.T.);
#2899=ORIENTED_EDGE('',*,*,#2216,.F.);
#2900=ORIENTED_EDGE('',*,*,#2285,.T.);
#2901=ORIENTED_EDGE('',*,*,#2260,.F.);
#2902=ORIENTED_EDGE('',*,*,#2286,.T.);
#2903=ORIENTED_EDGE('',*,*,#2267,.F.);
#2904=ORIENTED_EDGE('',*,*,#2287,.F.);
#2905=ORIENTED_EDGE('',*,*,#2288,.F.);
#2906=ORIENTED_EDGE('',*,*,#2289,.F.);
#2907=ORIENTED_EDGE('',*,*,#2290,.F.);
#2908=ORIENTED_EDGE('',*,*,#2278,.F.);
#2909=ORIENTED_EDGE('',*,*,#2291,.F.);
#2910=ORIENTED_EDGE('',*,*,#2292,.F.);
#2911=ORIENTED_EDGE('',*,*,#2293,.F.);
#2912=ORIENTED_EDGE('',*,*,#2294,.F.);
#2913=ORIENTED_EDGE('',*,*,#2295,.F.);
#2914=ORIENTED_EDGE('',*,*,#2296,.T.);
#2915=ORIENTED_EDGE('',*,*,#2264,.F.);
#2916=ORIENTED_EDGE('',*,*,#2297,.F.);
#2917=ORIENTED_EDGE('',*,*,#2206,.T.);
#2918=ORIENTED_EDGE('',*,*,#2209,.T.);
#2919=ORIENTED_EDGE('',*,*,#2290,.T.);
#2920=ORIENTED_EDGE('',*,*,#2298,.F.);
#2921=ORIENTED_EDGE('',*,*,#2249,.F.);
#2922=ORIENTED_EDGE('',*,*,#2279,.T.);
#2923=ORIENTED_EDGE('',*,*,#2289,.T.);
#2924=ORIENTED_EDGE('',*,*,#2299,.F.);
#2925=ORIENTED_EDGE('',*,*,#2250,.F.);
#2926=ORIENTED_EDGE('',*,*,#2298,.T.);
#2927=ORIENTED_EDGE('',*,*,#2288,.T.);
#2928=ORIENTED_EDGE('',*,*,#2300,.F.);
#2929=ORIENTED_EDGE('',*,*,#2251,.F.);
#2930=ORIENTED_EDGE('',*,*,#2299,.T.);
#2931=ORIENTED_EDGE('',*,*,#2287,.T.);
#2932=ORIENTED_EDGE('',*,*,#2269,.F.);
#2933=ORIENTED_EDGE('',*,*,#2252,.F.);
#2934=ORIENTED_EDGE('',*,*,#2300,.T.);
#2935=ORIENTED_EDGE('',*,*,#2235,.F.);
#2936=ORIENTED_EDGE('',*,*,#2301,.F.);
#2937=ORIENTED_EDGE('',*,*,#2295,.T.);
#2938=ORIENTED_EDGE('',*,*,#2302,.F.);
#2939=ORIENTED_EDGE('',*,*,#2294,.T.);
#2940=ORIENTED_EDGE('',*,*,#2303,.F.);
#2941=ORIENTED_EDGE('',*,*,#2236,.F.);
#2942=ORIENTED_EDGE('',*,*,#2302,.T.);
#2943=ORIENTED_EDGE('',*,*,#2293,.T.);
#2944=ORIENTED_EDGE('',*,*,#2304,.F.);
#2945=ORIENTED_EDGE('',*,*,#2237,.F.);
#2946=ORIENTED_EDGE('',*,*,#2303,.T.);
#2947=ORIENTED_EDGE('',*,*,#2292,.T.);
#2948=ORIENTED_EDGE('',*,*,#2305,.F.);
#2949=ORIENTED_EDGE('',*,*,#2238,.F.);
#2950=ORIENTED_EDGE('',*,*,#2304,.T.);
#2951=ORIENTED_EDGE('',*,*,#2291,.T.);
#2952=ORIENTED_EDGE('',*,*,#2277,.F.);
#2953=ORIENTED_EDGE('',*,*,#2239,.F.);
#2954=ORIENTED_EDGE('',*,*,#2305,.T.);
#2955=ORIENTED_EDGE('',*,*,#2306,.T.);
#2956=ORIENTED_EDGE('',*,*,#2242,.F.);
#2957=ORIENTED_EDGE('',*,*,#2307,.F.);
#2958=ORIENTED_EDGE('',*,*,#2275,.T.);
#2959=ORIENTED_EDGE('',*,*,#2276,.T.);
#2960=ORIENTED_EDGE('',*,*,#2307,.T.);
#2961=ORIENTED_EDGE('',*,*,#2241,.T.);
#2962=ORIENTED_EDGE('',*,*,#2274,.F.);
#2963=ORIENTED_EDGE('',*,*,#2243,.F.);
#2964=ORIENTED_EDGE('',*,*,#2306,.F.);
#2965=ORIENTED_EDGE('',*,*,#2308,.F.);
#2966=ORIENTED_EDGE('',*,*,#2272,.F.);
#2967=ORIENTED_EDGE('',*,*,#2309,.T.);
#2968=ORIENTED_EDGE('',*,*,#2246,.T.);
#2969=ORIENTED_EDGE('',*,*,#2271,.F.);
#2970=ORIENTED_EDGE('',*,*,#2247,.F.);
#2971=ORIENTED_EDGE('',*,*,#2309,.F.);
#2972=ORIENTED_EDGE('',*,*,#2273,.T.);
#2973=ORIENTED_EDGE('',*,*,#2308,.T.);
#2974=ORIENTED_EDGE('',*,*,#2245,.T.);
#2975=ORIENTED_EDGE('',*,*,#2266,.F.);
#2976=ORIENTED_EDGE('',*,*,#2232,.T.);
#2977=ORIENTED_EDGE('',*,*,#2268,.T.);
#2978=ORIENTED_EDGE('',*,*,#2286,.F.);
#2979=ORIENTED_EDGE('',*,*,#2301,.T.);
#2980=ORIENTED_EDGE('',*,*,#2234,.F.);
#2981=ORIENTED_EDGE('',*,*,#2265,.F.);
#2982=ORIENTED_EDGE('',*,*,#2296,.F.);
#2983=ORIENTED_EDGE('',*,*,#2310,.F.);
#2984=ORIENTED_EDGE('',*,*,#2311,.T.);
#2985=ORIENTED_EDGE('',*,*,#2202,.T.);
#2986=ORIENTED_EDGE('',*,*,#2312,.T.);
#2987=ORIENTED_EDGE('',*,*,#2313,.F.);
#2988=ORIENTED_EDGE('',*,*,#2297,.T.);
#2989=ORIENTED_EDGE('',*,*,#2314,.F.);
#2990=ORIENTED_EDGE('',*,*,#2315,.T.);
#2991=ORIENTED_EDGE('',*,*,#2316,.T.);
#2992=ORIENTED_EDGE('',*,*,#2317,.T.);
#2993=ORIENTED_EDGE('',*,*,#2318,.F.);
#2994=ORIENTED_EDGE('',*,*,#2200,.F.);
#2995=ORIENTED_EDGE('',*,*,#2262,.T.);
#2996=ORIENTED_EDGE('',*,*,#2319,.F.);
#2997=ORIENTED_EDGE('',*,*,#2316,.F.);
#2998=ORIENTED_EDGE('',*,*,#2320,.T.);
#2999=ORIENTED_EDGE('',*,*,#2313,.T.);
#3000=ORIENTED_EDGE('',*,*,#2321,.T.);
#3001=ORIENTED_EDGE('',*,*,#2317,.F.);
#3002=ORIENTED_EDGE('',*,*,#2319,.T.);
#3003=ORIENTED_EDGE('',*,*,#2261,.T.);
#3004=ORIENTED_EDGE('',*,*,#2315,.F.);
#3005=ORIENTED_EDGE('',*,*,#2322,.T.);
#3006=ORIENTED_EDGE('',*,*,#2310,.T.);
#3007=ORIENTED_EDGE('',*,*,#2263,.F.);
#3008=ORIENTED_EDGE('',*,*,#2320,.F.);
#3009=ORIENTED_EDGE('',*,*,#2322,.F.);
#3010=ORIENTED_EDGE('',*,*,#2314,.T.);
#3011=ORIENTED_EDGE('',*,*,#2203,.T.);
#3012=ORIENTED_EDGE('',*,*,#2311,.F.);
#3013=ORIENTED_EDGE('',*,*,#2282,.F.);
#3014=ORIENTED_EDGE('',*,*,#2281,.F.);
#3015=ORIENTED_EDGE('',*,*,#2211,.F.);
#3016=ORIENTED_EDGE('',*,*,#2285,.F.);
#3017=ORIENTED_EDGE('',*,*,#2215,.F.);
#3018=ORIENTED_EDGE('',*,*,#2284,.F.);
#3019=ORIENTED_EDGE('',*,*,#2219,.F.);
#3020=ORIENTED_EDGE('',*,*,#2270,.F.);
#3021=ORIENTED_EDGE('',*,*,#2225,.F.);
#3022=ORIENTED_EDGE('',*,*,#2283,.F.);
#3023=ORIENTED_EDGE('',*,*,#2228,.F.);
#3024=ORIENTED_EDGE('',*,*,#2186,.F.);
#3025=ORIENTED_EDGE('',*,*,#2231,.F.);
#3026=ORIENTED_EDGE('',*,*,#2321,.F.);
#3027=ORIENTED_EDGE('',*,*,#2312,.F.);
#3028=ORIENTED_EDGE('',*,*,#2201,.T.);
#3029=ORIENTED_EDGE('',*,*,#2318,.T.);
#3030=ORIENTED_EDGE('',*,*,#2197,.T.);
#3031=ORIENTED_EDGE('',*,*,#2192,.T.);
#3902=TOROIDAL_SURFACE('',#4252,39.2915026221292,8.);
#3903=TOROIDAL_SURFACE('',#4257,4.00000000000002,1.);
#3904=TOROIDAL_SURFACE('',#4263,4.00000000000002,1.);
#3921=ADVANCED_FACE('',(#1086),#3902,.F.);
#3922=ADVANCED_FACE('',(#1087),#3903,.T.);
#3923=ADVANCED_FACE('',(#1088),#1007,.T.);
#3924=ADVANCED_FACE('',(#1089),#3904,.T.);
#3925=ADVANCED_FACE('',(#1090),#1008,.T.);
#3926=ADVANCED_FACE('',(#1091),#1009,.F.);
#3927=ADVANCED_FACE('',(#1092),#1010,.F.);
#3928=ADVANCED_FACE('',(#1093),#1011,.F.);
#3929=ADVANCED_FACE('',(#1094),#1012,.F.);
#3930=ADVANCED_FACE('',(#1095),#1013,.F.);
#3931=ADVANCED_FACE('',(#1096),#1014,.F.);
#3932=ADVANCED_FACE('',(#1097),#1015,.T.);
#3933=ADVANCED_FACE('',(#1098),#1016,.T.);
#3934=ADVANCED_FACE('',(#1099),#1017,.T.);
#3935=ADVANCED_FACE('',(#1100,#112,#113,#114,#115),#159,.T.);
#3936=ADVANCED_FACE('',(#1101),#160,.F.);
#3937=ADVANCED_FACE('',(#1102),#161,.T.);
#3938=ADVANCED_FACE('',(#1103),#162,.F.);
#3939=ADVANCED_FACE('',(#1104,#116),#163,.F.);
#3940=ADVANCED_FACE('',(#1105),#164,.F.);
#3941=ADVANCED_FACE('',(#1106),#103,.T.);
#3942=ADVANCED_FACE('',(#1107),#165,.F.);
#3943=ADVANCED_FACE('',(#1108),#166,.F.);
#3944=ADVANCED_FACE('',(#1109),#167,.F.);
#3945=ADVANCED_FACE('',(#1110,#117,#118),#168,.F.);
#3946=ADVANCED_FACE('',(#1111),#169,.F.);
#3947=ADVANCED_FACE('',(#1112),#170,.F.);
#3948=ADVANCED_FACE('',(#1113),#1018,.T.);
#3949=ADVANCED_FACE('',(#1114),#171,.F.);
#3950=ADVANCED_FACE('',(#1115),#172,.F.);
#3951=ADVANCED_FACE('',(#1116),#173,.F.);
#3952=ADVANCED_FACE('',(#1117),#1019,.T.);
#3953=ADVANCED_FACE('',(#1118),#174,.F.);
#3954=ADVANCED_FACE('',(#1119),#175,.F.);
#3955=ADVANCED_FACE('',(#1120),#176,.F.);
#3956=ADVANCED_FACE('',(#1121),#177,.F.);
#3957=ADVANCED_FACE('',(#1122),#178,.T.);
#3958=ADVANCED_FACE('',(#1123),#179,.T.);
#3959=ADVANCED_FACE('',(#1124),#180,.F.);
#3960=ADVANCED_FACE('',(#1125),#181,.T.);
#3961=ADVANCED_FACE('',(#1126),#182,.F.);
#3962=ADVANCED_FACE('',(#1127),#183,.F.);
#3963=ADVANCED_FACE('',(#1128),#184,.F.);
#3964=ADVANCED_FACE('',(#1129),#185,.T.);
#3965=ADVANCED_FACE('',(#1130),#186,.F.);
#3966=ADVANCED_FACE('',(#1131),#187,.F.);
#3967=ADVANCED_FACE('',(#1132),#188,.F.);
#3968=ADVANCED_FACE('',(#1133),#189,.F.);
#3969=ADVANCED_FACE('',(#1134),#190,.F.);
#3970=ADVANCED_FACE('',(#1135),#191,.F.);
#3971=ADVANCED_FACE('',(#1136),#192,.F.);
#3972=ADVANCED_FACE('',(#1137),#193,.F.);
#4164=CLOSED_SHELL('',(#3921,#3922,#3923,#3924,#3925,#3926,#3927,#3928,
#3929,#3930,#3931,#3932,#3933,#3934,#3935,#3936,#3937,#3938,#3939,#3940,
#3941,#3942,#3943,#3944,#3945,#3946,#3947,#3948,#3949,#3950,#3951,#3952,
#3953,#3954,#3955,#3956,#3957,#3958,#3959,#3960,#3961,#3962,#3963,#3964,
#3965,#3966,#3967,#3968,#3969,#3970,#3971,#3972));
#4251=AXIS2_PLACEMENT_3D('',#5999,#4716,#4717);
#4252=AXIS2_PLACEMENT_3D('',#6000,#4718,#4719);
#4253=AXIS2_PLACEMENT_3D('',#6003,#4720,#4721);
#4254=AXIS2_PLACEMENT_3D('',#6005,#4722,#4723);
#4255=AXIS2_PLACEMENT_3D('',#6007,#4724,#4725);
#4256=AXIS2_PLACEMENT_3D('',#6008,#4726,#4727);
#4257=AXIS2_PLACEMENT_3D('',#6009,#4728,#4729);
#4258=AXIS2_PLACEMENT_3D('',#6011,#4730,#4731);
#4259=AXIS2_PLACEMENT_3D('',#6013,#4732,#4733);
#4260=AXIS2_PLACEMENT_3D('',#6014,#4734,#4735);
#4261=AXIS2_PLACEMENT_3D('',#6015,#4736,#4737);
#4262=AXIS2_PLACEMENT_3D('',#6017,#4738,#4739);
#4263=AXIS2_PLACEMENT_3D('',#6019,#4741,#4742);
#4264=AXIS2_PLACEMENT_3D('',#6021,#4743,#4744);
#4265=AXIS2_PLACEMENT_3D('',#6023,#4745,#4746);
#4266=AXIS2_PLACEMENT_3D('',#6024,#4747,#4748);
#4267=AXIS2_PLACEMENT_3D('',#6025,#4749,#4750);
#4268=AXIS2_PLACEMENT_3D('',#6027,#4751,#4752);
#4269=AXIS2_PLACEMENT_3D('',#6029,#4754,#4755);
#4270=AXIS2_PLACEMENT_3D('',#6032,#4756,#4757);
#4271=AXIS2_PLACEMENT_3D('',#6036,#4759,#4760);
#4272=AXIS2_PLACEMENT_3D('',#6038,#4762,#4763);
#4273=AXIS2_PLACEMENT_3D('',#6040,#4764,#4765);
#4274=AXIS2_PLACEMENT_3D('',#6043,#4767,#4768);
#4275=AXIS2_PLACEMENT_3D('',#6044,#4769,#4770);
#4276=AXIS2_PLACEMENT_3D('',#6046,#4771,#4772);
#4277=AXIS2_PLACEMENT_3D('',#6049,#4774,#4775);
#4278=AXIS2_PLACEMENT_3D('',#6050,#4776,#4777);
#4279=AXIS2_PLACEMENT_3D('',#6053,#4778,#4779);
#4280=AXIS2_PLACEMENT_3D('',#6057,#4781,#4782);
#4281=AXIS2_PLACEMENT_3D('',#6059,#4784,#4785);
#4282=AXIS2_PLACEMENT_3D('',#6062,#4786,#4787);
#4283=AXIS2_PLACEMENT_3D('',#6066,#4789,#4790);
#4284=AXIS2_PLACEMENT_3D('',#6068,#4792,#4793);
#4285=AXIS2_PLACEMENT_3D('',#6071,#4794,#4795);
#4286=AXIS2_PLACEMENT_3D('',#6075,#4797,#4798);
#4287=AXIS2_PLACEMENT_3D('',#6077,#4800,#4801);
#4288=AXIS2_PLACEMENT_3D('',#6080,#4802,#4803);
#4289=AXIS2_PLACEMENT_3D('',#6084,#4805,#4806);
#4290=AXIS2_PLACEMENT_3D('',#6086,#4808,#4809);
#4291=AXIS2_PLACEMENT_3D('',#6089,#4810,#4811);
#4292=AXIS2_PLACEMENT_3D('',#6092,#4814,#4815);
#4293=AXIS2_PLACEMENT_3D('',#6096,#4817,#4818);
#4294=AXIS2_PLACEMENT_3D('',#6098,#4820,#4821);
#4295=AXIS2_PLACEMENT_3D('',#6111,#4827,#4828);
#4296=AXIS2_PLACEMENT_3D('',#6139,#4842,#4843);
#4297=AXIS2_PLACEMENT_3D('',#6143,#4846,#4847);
#4298=AXIS2_PLACEMENT_3D('',#6151,#4854,#4855);
#4299=AXIS2_PLACEMENT_3D('',#6165,#4863,#4864);
#4300=AXIS2_PLACEMENT_3D('',#6171,#4868,#4869);
#4301=AXIS2_PLACEMENT_3D('',#6188,#4880,#4881);
#4302=AXIS2_PLACEMENT_3D('',#6190,#4882,#4883);
#4303=AXIS2_PLACEMENT_3D('',#6192,#4885,#4886);
#4304=AXIS2_PLACEMENT_3D('',#6194,#4888,#4889);
#4305=AXIS2_PLACEMENT_3D('',#6196,#4891,#4892);
#4306=AXIS2_PLACEMENT_3D('',#6198,#4894,#4895);
#4307=AXIS2_PLACEMENT_3D('',#6200,#4897,#4898);
#4308=AXIS2_PLACEMENT_3D('',#6205,#4901,#4902);
#4309=AXIS2_PLACEMENT_3D('',#6214,#4907,#4908);
#4310=AXIS2_PLACEMENT_3D('',#6221,#4913,#4914);
#4311=AXIS2_PLACEMENT_3D('',#6223,#4916,#4917);
#4312=AXIS2_PLACEMENT_3D('',#6225,#4919,#4920);
#4313=AXIS2_PLACEMENT_3D('',#6227,#4922,#4923);
#4314=AXIS2_PLACEMENT_3D('',#6228,#4924,#4925);
#4315=AXIS2_PLACEMENT_3D('',#6231,#4928,#4929);
#4316=AXIS2_PLACEMENT_3D('',#6233,#4931,#4932);
#4317=AXIS2_PLACEMENT_3D('',#6235,#4934,#4935);
#4318=AXIS2_PLACEMENT_3D('',#6237,#4937,#4938);
#4319=AXIS2_PLACEMENT_3D('',#6238,#4939,#4940);
#4320=AXIS2_PLACEMENT_3D('',#6241,#4943,#4944);
#4321=AXIS2_PLACEMENT_3D('',#6242,#4945,#4946);
#4322=AXIS2_PLACEMENT_3D('',#6243,#4947,#4948);
#4323=AXIS2_PLACEMENT_3D('',#6246,#4951,#4952);
#4324=AXIS2_PLACEMENT_3D('',#6247,#4953,#4954);
#4325=AXIS2_PLACEMENT_3D('',#6248,#4955,#4956);
#4326=AXIS2_PLACEMENT_3D('',#6249,#4957,#4958);
#4327=AXIS2_PLACEMENT_3D('',#6250,#4959,#4960);
#4328=AXIS2_PLACEMENT_3D('',#6257,#4965,#4966);
#4329=AXIS2_PLACEMENT_3D('',#6267,#4972,#4973);
#4330=AXIS2_PLACEMENT_3D('',#6270,#4976,#4977);
#4331=AXIS2_PLACEMENT_3D('',#6272,#4979,#4980);
#4332=AXIS2_PLACEMENT_3D('',#6274,#4982,#4983);
#4333=AXIS2_PLACEMENT_3D('',#6275,#4984,#4985);
#4334=AXIS2_PLACEMENT_3D('',#6276,#4986,#4987);
#4335=AXIS2_PLACEMENT_3D('',#6277,#4988,#4989);
#4336=AXIS2_PLACEMENT_3D('',#6278,#4990,#4991);
#4716=DIRECTION('axis',(0.,0.,1.));
#4717=DIRECTION('refdir',(1.,0.,0.));
#4718=DIRECTION('center_axis',(0.,0.,1.));
#4719=DIRECTION('ref_axis',(1.,0.,0.));
#4720=DIRECTION('center_axis',(-1.,0.,0.));
#4721=DIRECTION('ref_axis',(0.,0.,-1.));
#4722=DIRECTION('center_axis',(0.,0.,1.));
#4723=DIRECTION('ref_axis',(1.,0.,0.));
#4724=DIRECTION('center_axis',(-1.,0.,0.));
#4725=DIRECTION('ref_axis',(0.,-1.73472347597681E-15,-1.));
#4726=DIRECTION('center_axis',(0.,0.,1.));
#4727=DIRECTION('ref_axis',(1.,0.,0.));
#4728=DIRECTION('center_axis',(-1.,0.,0.));
#4729=DIRECTION('ref_axis',(0.,0.,1.));
#4730=DIRECTION('center_axis',(-1.,0.,0.));
#4731=DIRECTION('ref_axis',(0.,0.,1.));
#4732=DIRECTION('center_axis',(0.,-1.,0.));
#4733=DIRECTION('ref_axis',(0.,0.,-1.));
#4734=DIRECTION('center_axis',(1.,0.,0.));
#4735=DIRECTION('ref_axis',(0.,0.,1.));
#4736=DIRECTION('center_axis',(-1.,0.,0.));
#4737=DIRECTION('ref_axis',(0.,0.,1.));
#4738=DIRECTION('center_axis',(-1.,0.,0.));
#4739=DIRECTION('ref_axis',(0.,0.,-1.));
#4740=DIRECTION('',(1.,0.,0.));
#4741=DIRECTION('center_axis',(-1.,0.,0.));
#4742=DIRECTION('ref_axis',(0.,0.,1.));
#4743=DIRECTION('center_axis',(-1.,0.,0.));
#4744=DIRECTION('ref_axis',(0.,0.,1.));
#4745=DIRECTION('center_axis',(0.,-1.,0.));
#4746=DIRECTION('ref_axis',(0.,0.,-1.));
#4747=DIRECTION('center_axis',(1.,0.,0.));
#4748=DIRECTION('ref_axis',(0.,0.,1.));
#4749=DIRECTION('center_axis',(-1.,0.,0.));
#4750=DIRECTION('ref_axis',(0.,0.,1.));
#4751=DIRECTION('center_axis',(1.,0.,0.));
#4752=DIRECTION('ref_axis',(0.,0.,-1.));
#4753=DIRECTION('',(1.,0.,0.));
#4754=DIRECTION('center_axis',(0.,0.,1.));
#4755=DIRECTION('ref_axis',(1.,0.,0.));
#4756=DIRECTION('center_axis',(0.,0.,-1.));
#4757=DIRECTION('ref_axis',(-1.,0.,0.));
#4758=DIRECTION('',(0.,0.,-1.));
#4759=DIRECTION('center_axis',(0.,0.,-1.));
#4760=DIRECTION('ref_axis',(-1.,0.,0.));
#4761=DIRECTION('',(0.,0.,1.));
#4762=DIRECTION('center_axis',(-1.,0.,0.));
#4763=DIRECTION('ref_axis',(0.,0.,1.));
#4764=DIRECTION('center_axis',(1.,0.,0.));
#4765=DIRECTION('ref_axis',(0.,0.,1.));
#4766=DIRECTION('',(-1.,0.,0.));
#4767=DIRECTION('center_axis',(1.,0.,0.));
#4768=DIRECTION('ref_axis',(0.,0.,1.));
#4769=DIRECTION('center_axis',(-1.,0.,0.));
#4770=DIRECTION('ref_axis',(0.,0.,1.));
#4771=DIRECTION('center_axis',(1.,0.,0.));
#4772=DIRECTION('ref_axis',(0.,0.,-1.));
#4773=DIRECTION('',(-1.,0.,0.));
#4774=DIRECTION('center_axis',(1.,0.,0.));
#4775=DIRECTION('ref_axis',(0.,0.,-1.));
#4776=DIRECTION('center_axis',(0.,0.,1.));
#4777=DIRECTION('ref_axis',(1.,0.,0.));
#4778=DIRECTION('center_axis',(0.,0.,1.));
#4779=DIRECTION('ref_axis',(1.,0.,0.));
#4780=DIRECTION('',(0.,0.,1.));
#4781=DIRECTION('center_axis',(0.,0.,1.));
#4782=DIRECTION('ref_axis',(1.,0.,0.));
#4783=DIRECTION('',(0.,0.,-1.));
#4784=DIRECTION('center_axis',(0.,0.,1.));
#4785=DIRECTION('ref_axis',(1.,0.,0.));
#4786=DIRECTION('center_axis',(0.,0.,1.));
#4787=DIRECTION('ref_axis',(1.,0.,0.));
#4788=DIRECTION('',(0.,0.,1.));
#4789=DIRECTION('center_axis',(0.,0.,1.));
#4790=DIRECTION('ref_axis',(1.,0.,0.));
#4791=DIRECTION('',(0.,0.,-1.));
#4792=DIRECTION('center_axis',(0.,0.,1.));
#4793=DIRECTION('ref_axis',(1.,0.,0.));
#4794=DIRECTION('center_axis',(0.,0.,1.));
#4795=DIRECTION('ref_axis',(1.,0.,0.));
#4796=DIRECTION('',(0.,0.,1.));
#4797=DIRECTION('center_axis',(0.,0.,1.));
#4798=DIRECTION('ref_axis',(1.,0.,0.));
#4799=DIRECTION('',(0.,0.,-1.));
#4800=DIRECTION('center_axis',(0.,0.,1.));
#4801=DIRECTION('ref_axis',(1.,0.,0.));
#4802=DIRECTION('center_axis',(0.,0.,1.));
#4803=DIRECTION('ref_axis',(1.,0.,0.));
#4804=DIRECTION('',(0.,0.,1.));
#4805=DIRECTION('center_axis',(0.,0.,1.));
#4806=DIRECTION('ref_axis',(1.,0.,0.));
#4807=DIRECTION('',(0.,0.,-1.));
#4808=DIRECTION('center_axis',(0.,0.,1.));
#4809=DIRECTION('ref_axis',(1.,0.,0.));
#4810=DIRECTION('center_axis',(0.,0.,1.));
#4811=DIRECTION('ref_axis',(1.,0.,0.));
#4812=DIRECTION('',(0.,0.,1.));
#4813=DIRECTION('',(0.,0.,-1.));
#4814=DIRECTION('center_axis',(0.,0.,1.));
#4815=DIRECTION('ref_axis',(1.,0.,0.));
#4816=DIRECTION('',(0.,0.,1.));
#4817=DIRECTION('center_axis',(0.,0.,1.));
#4818=DIRECTION('ref_axis',(1.,0.,0.));
#4819=DIRECTION('',(0.,0.,-1.));
#4820=DIRECTION('center_axis',(1.,0.,0.));
#4821=DIRECTION('ref_axis',(0.,0.,-1.));
#4822=DIRECTION('',(0.,0.,-1.));
#4823=DIRECTION('',(-8.67361737988404E-17,-1.,0.));
#4824=DIRECTION('',(0.,0.,-1.));
#4825=DIRECTION('',(0.,1.,0.));
#4826=DIRECTION('',(0.,0.672272926960032,0.740303391641961));
#4827=DIRECTION('center_axis',(1.,0.,0.));
#4828=DIRECTION('ref_axis',(0.,0.,1.));
#4829=DIRECTION('',(0.,-0.669715115850366,0.742618114242799));
#4830=DIRECTION('',(0.,0.,1.));
#4831=DIRECTION('',(0.,-1.,0.));
#4832=DIRECTION('',(0.,0.,1.));
#4833=DIRECTION('',(0.,-1.,0.));
#4834=DIRECTION('',(0.,0.,1.));
#4835=DIRECTION('',(0.,-1.,0.));
#4836=DIRECTION('',(0.,0.,1.));
#4837=DIRECTION('',(0.,1.,0.));
#4838=DIRECTION('',(0.,0.,1.));
#4839=DIRECTION('',(0.,-1.,0.));
#4840=DIRECTION('',(0.,0.,-1.));
#4841=DIRECTION('',(0.,-0.669715115850366,-0.742618114242799));
#4842=DIRECTION('center_axis',(1.,0.,0.));
#4843=DIRECTION('ref_axis',(0.,0.,-1.));
#4844=DIRECTION('',(0.,0.672272926960032,-0.740303391641961));
#4845=DIRECTION('',(0.,1.,0.));
#4846=DIRECTION('center_axis',(1.,0.,0.));
#4847=DIRECTION('ref_axis',(0.,0.,-1.));
#4848=DIRECTION('',(0.,-0.175790638483658,0.984427575508482));
#4849=DIRECTION('',(0.,-1.,0.));
#4850=DIRECTION('',(0.,1.,0.));
#4851=DIRECTION('',(0.,-1.,0.));
#4852=DIRECTION('',(0.,-1.,0.));
#4853=DIRECTION('',(0.,-1.,0.));
#4854=DIRECTION('center_axis',(0.,0.,-1.));
#4855=DIRECTION('ref_axis',(-1.,0.,0.));
#4856=DIRECTION('',(0.,1.,0.));
#4857=DIRECTION('',(-1.,0.,0.));
#4858=DIRECTION('',(0.,-1.,0.));
#4859=DIRECTION('',(-1.,1.50845519650157E-16,0.));
#4860=DIRECTION('',(0.,1.,0.));
#4861=DIRECTION('',(1.,-2.89120579329468E-16,0.));
#4862=DIRECTION('',(-1.,0.,0.));
#4863=DIRECTION('center_axis',(0.,0.,1.));
#4864=DIRECTION('ref_axis',(1.,0.,0.));
#4865=DIRECTION('',(0.,1.,0.));
#4866=DIRECTION('',(-1.,0.,0.));
#4867=DIRECTION('',(-1.,0.,0.));
#4868=DIRECTION('center_axis',(0.,0.,1.));
#4869=DIRECTION('ref_axis',(1.,0.,0.));
#4870=DIRECTION('',(0.,1.,0.));
#4871=DIRECTION('',(1.,0.,6.93889390390723E-16));
#4872=DIRECTION('',(0.,1.,0.));
#4873=DIRECTION('',(1.,0.,6.93889390390723E-16));
#4874=DIRECTION('',(1.,0.,6.93889390390723E-16));
#4875=DIRECTION('',(0.,-1.,0.));
#4876=DIRECTION('',(1.,0.,6.93889390390723E-16));
#4877=DIRECTION('',(-1.,0.,0.));
#4878=DIRECTION('',(0.,-1.,0.));
#4879=DIRECTION('',(-1.,0.,0.));
#4880=DIRECTION('center_axis',(0.,0.,-1.));
#4881=DIRECTION('ref_axis',(-1.,0.,0.));
#4882=DIRECTION('center_axis',(0.,0.,1.));
#4883=DIRECTION('ref_axis',(1.,0.,0.));
#4884=DIRECTION('',(0.,-1.,0.));
#4885=DIRECTION('center_axis',(0.,0.,-1.));
#4886=DIRECTION('ref_axis',(1.,1.22464679914735E-16,0.));
#4887=DIRECTION('',(0.,-0.175790638483658,-0.984427575508482));
#4888=DIRECTION('center_axis',(0.,0.,-1.));
#4889=DIRECTION('ref_axis',(-1.,0.,0.));
#4890=DIRECTION('',(0.,-1.,0.));
#4891=DIRECTION('center_axis',(0.,0.,-1.));
#4892=DIRECTION('ref_axis',(-1.,0.,0.));
#4893=DIRECTION('',(0.,-1.,0.));
#4894=DIRECTION('center_axis',(0.,0.,-1.));
#4895=DIRECTION('ref_axis',(-1.,0.,0.));
#4896=DIRECTION('',(0.,-1.,0.));
#4897=DIRECTION('center_axis',(1.,0.,0.));
#4898=DIRECTION('ref_axis',(0.,0.,-1.));
#4899=DIRECTION('',(0.,0.,-1.));
#4900=DIRECTION('',(0.,0.672272926960032,-0.740303391641961));
#4901=DIRECTION('center_axis',(1.,0.,0.));
#4902=DIRECTION('ref_axis',(0.,0.,-1.));
#4903=DIRECTION('',(0.,-0.669715115850366,-0.742618114242799));
#4904=DIRECTION('',(0.,0.,-1.));
#4905=DIRECTION('',(0.,0.,1.));
#4906=DIRECTION('',(0.,-0.669715115850366,0.742618114242799));
#4907=DIRECTION('center_axis',(1.,0.,0.));
#4908=DIRECTION('ref_axis',(0.,0.,1.));
#4909=DIRECTION('',(0.,0.672272926960032,0.740303391641961));
#4910=DIRECTION('',(0.,1.,0.));
#4911=DIRECTION('',(0.,0.,1.));
#4912=DIRECTION('',(0.,1.,0.));
#4913=DIRECTION('center_axis',(0.,1.,0.));
#4914=DIRECTION('ref_axis',(0.,0.,1.));
#4915=DIRECTION('',(-1.,0.,0.));
#4916=DIRECTION('center_axis',(0.,0.742618114242799,-0.669715115850366));
#4917=DIRECTION('ref_axis',(0.,0.669715115850366,0.742618114242799));
#4918=DIRECTION('',(-1.,0.,0.));
#4919=DIRECTION('center_axis',(-1.,0.,0.));
#4920=DIRECTION('ref_axis',(0.,0.,1.));
#4921=DIRECTION('',(-1.,0.,0.));
#4922=DIRECTION('center_axis',(0.,0.740303391641961,0.672272926960032));
#4923=DIRECTION('ref_axis',(0.,-0.672272926960032,0.740303391641961));
#4924=DIRECTION('center_axis',(0.,0.,1.));
#4925=DIRECTION('ref_axis',(1.,0.,0.));
#4926=DIRECTION('',(1.,-2.89120579329468E-16,0.));
#4927=DIRECTION('',(-1.,0.,0.));
#4928=DIRECTION('center_axis',(0.,-0.740303391641961,0.672272926960032));
#4929=DIRECTION('ref_axis',(0.,-0.672272926960032,-0.740303391641961));
#4930=DIRECTION('',(-1.,0.,0.));
#4931=DIRECTION('center_axis',(-1.,0.,0.));
#4932=DIRECTION('ref_axis',(0.,0.,1.));
#4933=DIRECTION('',(-1.,0.,0.));
#4934=DIRECTION('center_axis',(0.,-0.742618114242799,-0.669715115850366));
#4935=DIRECTION('ref_axis',(0.,0.669715115850366,-0.742618114242799));
#4936=DIRECTION('',(-1.,0.,0.));
#4937=DIRECTION('center_axis',(0.,-1.,0.));
#4938=DIRECTION('ref_axis',(0.,0.,-1.));
#4939=DIRECTION('center_axis',(-0.968938918897475,0.,0.247300164669968));
#4940=DIRECTION('ref_axis',(0.247300164669968,0.,0.968938918897475));
#4941=DIRECTION('',(-0.247300164669968,0.,-0.968938918897475));
#4942=DIRECTION('',(-0.247300164669968,0.,-0.968938918897475));
#4943=DIRECTION('center_axis',(0.,-1.,0.));
#4944=DIRECTION('ref_axis',(0.,0.,-1.));
#4945=DIRECTION('center_axis',(0.,-1.,0.));
#4946=DIRECTION('ref_axis',(0.,0.,-1.));
#4947=DIRECTION('center_axis',(0.968938918897475,0.,-0.247300164669968));
#4948=DIRECTION('ref_axis',(-0.247300164669968,0.,-0.968938918897475));
#4949=DIRECTION('',(-0.247300164669968,0.,-0.968938918897475));
#4950=DIRECTION('',(-0.247300164669968,0.,-0.968938918897475));
#4951=DIRECTION('center_axis',(0.,1.,0.));
#4952=DIRECTION('ref_axis',(0.,0.,-1.));
#4953=DIRECTION('center_axis',(0.,1.,0.));
#4954=DIRECTION('ref_axis',(0.,0.,-1.));
#4955=DIRECTION('center_axis',(0.,-1.,0.));
#4956=DIRECTION('ref_axis',(0.,0.,-1.));
#4957=DIRECTION('center_axis',(2.89120579329468E-16,1.,0.));
#4958=DIRECTION('ref_axis',(-1.,2.89120579329468E-16,0.));
#4959=DIRECTION('center_axis',(0.,0.,-1.));
#4960=DIRECTION('ref_axis',(-1.,0.,0.));
#4961=DIRECTION('',(1.,-1.50845519650157E-16,0.));
#4962=DIRECTION('',(0.,-1.,0.));
#4963=DIRECTION('',(0.,-1.,0.));
#4964=DIRECTION('',(-1.,0.,0.));
#4965=DIRECTION('center_axis',(0.,0.,-1.));
#4966=DIRECTION('ref_axis',(-1.,0.,0.));
#4967=DIRECTION('',(0.,-1.,0.));
#4968=DIRECTION('',(1.,-1.50845519650157E-16,0.));
#4969=DIRECTION('',(0.,-1.,0.));
#4970=DIRECTION('',(-1.,0.,0.));
#4971=DIRECTION('',(0.,-1.,0.));
#4972=DIRECTION('center_axis',(-1.,0.,0.));
#4973=DIRECTION('ref_axis',(0.,0.,1.));
#4974=DIRECTION('',(0.,0.,1.));
#4975=DIRECTION('',(0.,0.,1.));
#4976=DIRECTION('center_axis',(0.,1.,0.));
#4977=DIRECTION('ref_axis',(0.,0.,1.));
#4978=DIRECTION('',(0.,0.,-1.));
#4979=DIRECTION('center_axis',(-1.50845519650157E-16,-1.,0.));
#4980=DIRECTION('ref_axis',(1.,-1.50845519650157E-16,0.));
#4981=DIRECTION('',(0.,0.,1.));
#4982=DIRECTION('center_axis',(1.,0.,0.));
#4983=DIRECTION('ref_axis',(0.,0.,-1.));
#4984=DIRECTION('center_axis',(1.,0.,0.));
#4985=DIRECTION('ref_axis',(0.,0.,-1.));
#4986=DIRECTION('center_axis',(1.,0.,0.));
#4987=DIRECTION('ref_axis',(0.,0.,-1.));
#4988=DIRECTION('center_axis',(-1.,0.,0.));
#4989=DIRECTION('ref_axis',(0.,0.,1.));
#4990=DIRECTION('center_axis',(-1.,0.,0.));
#4991=DIRECTION('ref_axis',(0.,0.,1.));
#5999=CARTESIAN_POINT('',(0.,0.,0.));
#6000=CARTESIAN_POINT('Origin',(0.,0.,-50.));
#6001=CARTESIAN_POINT('',(0.,-34.,-44.));
#6002=CARTESIAN_POINT('',(0.,-34.,-56.));
#6003=CARTESIAN_POINT('Origin',(0.,-39.2915026221292,-50.));
#6004=CARTESIAN_POINT('',(0.,34.,-56.));
#6005=CARTESIAN_POINT('Origin',(0.,0.,-56.));
#6006=CARTESIAN_POINT('',(0.,34.,-44.));
#6007=CARTESIAN_POINT('Origin',(0.,39.2915026221292,-50.));
#6008=CARTESIAN_POINT('Origin',(0.,0.,-44.));
#6009=CARTESIAN_POINT('Origin',(33.,41.,-147.));
#6010=CARTESIAN_POINT('',(33.,41.,-152.));
#6011=CARTESIAN_POINT('Origin',(33.,41.,-147.));
#6012=CARTESIAN_POINT('',(34.,41.,-151.));
#6013=CARTESIAN_POINT('Origin',(33.,41.,-151.));
#6014=CARTESIAN_POINT('Origin',(34.,41.,-147.));
#6015=CARTESIAN_POINT('Origin',(34.,41.,-147.));
#6016=CARTESIAN_POINT('',(24.,41.,-152.));
#6017=CARTESIAN_POINT('Origin',(24.,41.,-147.));
#6018=CARTESIAN_POINT('',(34.,41.,-152.));
#6019=CARTESIAN_POINT('Origin',(33.,-41.,-147.));
#6020=CARTESIAN_POINT('',(33.,-41.,-152.));
#6021=CARTESIAN_POINT('Origin',(33.,-41.,-147.));
#6022=CARTESIAN_POINT('',(34.,-41.,-151.));
#6023=CARTESIAN_POINT('Origin',(33.,-41.,-151.));
#6024=CARTESIAN_POINT('Origin',(34.,-41.,-147.));
#6025=CARTESIAN_POINT('Origin',(34.,-41.,-147.));
#6026=CARTESIAN_POINT('',(24.,-41.,-152.));
#6027=CARTESIAN_POINT('Origin',(24.,-41.,-147.));
#6028=CARTESIAN_POINT('',(34.,-41.,-152.));
#6029=CARTESIAN_POINT('Origin',(0.,0.,-165.));
#6030=CARTESIAN_POINT('',(0.,5.,-165.));
#6031=CARTESIAN_POINT('',(0.,-5.,-165.));
#6032=CARTESIAN_POINT('Origin',(0.,0.,-165.));
#6033=CARTESIAN_POINT('',(0.,-5.,-153.));
#6034=CARTESIAN_POINT('',(0.,-5.,-165.));
#6035=CARTESIAN_POINT('',(0.,5.,-153.));
#6036=CARTESIAN_POINT('Origin',(0.,0.,-153.));
#6037=CARTESIAN_POINT('',(0.,5.,-165.));
#6038=CARTESIAN_POINT('Origin',(24.,-67.,-127.));
#6039=CARTESIAN_POINT('',(24.,-67.,-132.));
#6040=CARTESIAN_POINT('Origin',(24.,-67.,-127.));
#6041=CARTESIAN_POINT('',(16.,-67.,-132.));
#6042=CARTESIAN_POINT('',(24.,-67.,-132.));
#6043=CARTESIAN_POINT('Origin',(16.,-67.,-127.));
#6044=CARTESIAN_POINT('Origin',(24.,67.,-127.));
#6045=CARTESIAN_POINT('',(24.,67.,-132.));
#6046=CARTESIAN_POINT('Origin',(24.,67.,-127.));
#6047=CARTESIAN_POINT('',(16.,67.,-132.));
#6048=CARTESIAN_POINT('',(24.,67.,-132.));
#6049=CARTESIAN_POINT('Origin',(16.,67.,-127.));
#6050=CARTESIAN_POINT('Origin',(0.,0.,54.));
#6051=CARTESIAN_POINT('',(0.,-23.5,-46.));
#6052=CARTESIAN_POINT('',(0.,23.5,-46.));
#6053=CARTESIAN_POINT('Origin',(0.,0.,-46.));
#6054=CARTESIAN_POINT('',(0.,-23.5,-9.18183714823662E-16));
#6055=CARTESIAN_POINT('',(0.,-23.5,54.));
#6056=CARTESIAN_POINT('',(0.,23.5,0.));
#6057=CARTESIAN_POINT('Origin',(0.,0.,-9.18183714823662E-16));
#6058=CARTESIAN_POINT('',(0.,23.5,54.));
#6059=CARTESIAN_POINT('Origin',(0.,0.,54.));
#6060=CARTESIAN_POINT('',(0.,-22.,-63.));
#6061=CARTESIAN_POINT('',(0.,22.,-63.));
#6062=CARTESIAN_POINT('Origin',(0.,0.,-63.));
#6063=CARTESIAN_POINT('',(0.,-22.,-46.));
#6064=CARTESIAN_POINT('',(0.,-22.,54.));
#6065=CARTESIAN_POINT('',(0.,22.,-46.));
#6066=CARTESIAN_POINT('Origin',(0.,0.,-46.));
#6067=CARTESIAN_POINT('',(0.,22.,54.));
#6068=CARTESIAN_POINT('Origin',(0.,0.,54.));
#6069=CARTESIAN_POINT('',(0.,-15.,-71.));
#6070=CARTESIAN_POINT('',(0.,15.,-71.));
#6071=CARTESIAN_POINT('Origin',(0.,0.,-71.));
#6072=CARTESIAN_POINT('',(0.,-15.,-63.));
#6073=CARTESIAN_POINT('',(0.,-15.,54.));
#6074=CARTESIAN_POINT('',(0.,15.,-63.));
#6075=CARTESIAN_POINT('Origin',(0.,0.,-63.));
#6076=CARTESIAN_POINT('',(0.,15.,54.));
#6077=CARTESIAN_POINT('Origin',(0.,0.,54.));
#6078=CARTESIAN_POINT('',(0.,-55.,-71.));
#6079=CARTESIAN_POINT('',(0.,55.,-71.));
#6080=CARTESIAN_POINT('Origin',(0.,0.,-71.));
#6081=CARTESIAN_POINT('',(0.,55.,-63.));
#6082=CARTESIAN_POINT('',(0.,55.,54.));
#6083=CARTESIAN_POINT('',(0.,-55.,-63.));
#6084=CARTESIAN_POINT('Origin',(0.,0.,-63.));
#6085=CARTESIAN_POINT('',(0.,-55.,54.));
#6086=CARTESIAN_POINT('Origin',(0.,0.,54.));
#6087=CARTESIAN_POINT('',(0.,-34.,-63.));
#6088=CARTESIAN_POINT('',(0.,34.,-63.));
#6089=CARTESIAN_POINT('Origin',(0.,0.,-63.));
#6090=CARTESIAN_POINT('',(0.,34.,54.));
#6091=CARTESIAN_POINT('',(0.,-34.,54.));
#6092=CARTESIAN_POINT('Origin',(0.,0.,54.));
#6093=CARTESIAN_POINT('',(0.,34.,-14.));
#6094=CARTESIAN_POINT('',(0.,34.,54.));
#6095=CARTESIAN_POINT('',(0.,-34.,-14.));
#6096=CARTESIAN_POINT('Origin',(0.,0.,-14.));
#6097=CARTESIAN_POINT('',(0.,-34.,54.));
#6098=CARTESIAN_POINT('Origin',(24.,-67.,-127.));
#6099=CARTESIAN_POINT('',(24.,-20.,-153.));
#6100=CARTESIAN_POINT('',(24.,-20.,-165.));
#6101=CARTESIAN_POINT('',(24.,-20.,-153.));
#6102=CARTESIAN_POINT('',(24.,20.,-153.));
#6103=CARTESIAN_POINT('',(24.,-20.,-153.));
#6104=CARTESIAN_POINT('',(24.,20.,-165.));
#6105=CARTESIAN_POINT('',(24.,20.,-153.));
#6106=CARTESIAN_POINT('',(24.,46.,-165.));
#6107=CARTESIAN_POINT('',(24.,-46.,-165.));
#6108=CARTESIAN_POINT('',(24.,74.4030339164196,-133.7227292696));
#6109=CARTESIAN_POINT('',(24.,74.4030339164196,-133.7227292696));
#6110=CARTESIAN_POINT('',(24.,74.426181142428,-120.302848841496));
#6111=CARTESIAN_POINT('Origin',(24.,67.,-127.));
#6112=CARTESIAN_POINT('',(24.,48.,-91.));
#6113=CARTESIAN_POINT('',(24.,48.,-91.));
#6114=CARTESIAN_POINT('',(24.,48.,-71.));
#6115=CARTESIAN_POINT('',(24.,48.,-71.));
#6116=CARTESIAN_POINT('',(24.,29.,-71.));
#6117=CARTESIAN_POINT('',(24.,48.,-71.));
#6118=CARTESIAN_POINT('',(24.,29.,-149.3613646348));
#6119=CARTESIAN_POINT('',(24.,29.,-71.));
#6120=CARTESIAN_POINT('',(24.,21.,-149.3613646348));
#6121=CARTESIAN_POINT('',(24.,29.,-149.3613646348));
#6122=CARTESIAN_POINT('',(24.,21.,-71.));
#6123=CARTESIAN_POINT('',(24.,21.,-71.));
#6124=CARTESIAN_POINT('',(24.,-21.,-71.));
#6125=CARTESIAN_POINT('',(24.,48.,-71.));
#6126=CARTESIAN_POINT('',(24.,-21.,-149.3613646348));
#6127=CARTESIAN_POINT('',(24.,-21.,-71.));
#6128=CARTESIAN_POINT('',(24.,-29.,-149.3613646348));
#6129=CARTESIAN_POINT('',(24.,-29.,-149.3613646348));
#6130=CARTESIAN_POINT('',(24.,-29.,-71.));
#6131=CARTESIAN_POINT('',(24.,-29.,-71.));
#6132=CARTESIAN_POINT('',(24.,-48.,-71.));
#6133=CARTESIAN_POINT('',(24.,48.,-71.));
#6134=CARTESIAN_POINT('',(24.,-48.,-91.));
#6135=CARTESIAN_POINT('',(24.,-48.,-71.));
#6136=CARTESIAN_POINT('',(24.,-74.426181142428,-120.302848841496));
#6137=CARTESIAN_POINT('',(24.,-48.,-91.));
#6138=CARTESIAN_POINT('',(24.,-74.4030339164196,-133.7227292696));
#6139=CARTESIAN_POINT('Origin',(24.,-67.,-127.));
#6140=CARTESIAN_POINT('',(24.,-46.,-165.));
#6141=CARTESIAN_POINT('',(24.,-74.4030339164196,-133.7227292696));
#6142=CARTESIAN_POINT('',(24.,-46.,-165.));
#6143=CARTESIAN_POINT('Origin',(0.,93.,313.849585789117));
#6144=CARTESIAN_POINT('',(0.,31.5,6.12303176911193E-17));
#6145=CARTESIAN_POINT('',(0.,0.,176.4));
#6146=CARTESIAN_POINT('',(0.,55.,-63.));
#6147=CARTESIAN_POINT('',(0.,15.,-71.));
#6148=CARTESIAN_POINT('',(0.,22.,-63.));
#6149=CARTESIAN_POINT('',(0.,23.5,-46.));
#6150=CARTESIAN_POINT('',(0.,31.5,6.12303176911193E-17));
#6151=CARTESIAN_POINT('Origin',(-24.,20.,-153.));
#6152=CARTESIAN_POINT('',(16.,-20.,-153.));
#6153=CARTESIAN_POINT('',(16.,-19.,-153.));
#6154=CARTESIAN_POINT('',(16.,-67.,-153.));
#6155=CARTESIAN_POINT('',(23.,-19.,-153.));
#6156=CARTESIAN_POINT('',(23.,-19.,-153.));
#6157=CARTESIAN_POINT('',(23.,19.,-153.));
#6158=CARTESIAN_POINT('',(23.,19.,-153.));
#6159=CARTESIAN_POINT('',(16.,19.,-153.));
#6160=CARTESIAN_POINT('',(-24.,19.,-153.));
#6161=CARTESIAN_POINT('',(16.,20.,-153.));
#6162=CARTESIAN_POINT('',(16.,-67.,-153.));
#6163=CARTESIAN_POINT('',(-24.,20.,-153.));
#6164=CARTESIAN_POINT('',(-24.,-20.,-153.));
#6165=CARTESIAN_POINT('Origin',(24.,46.,-165.));
#6166=CARTESIAN_POINT('',(16.,-46.,-165.));
#6167=CARTESIAN_POINT('',(16.,-20.,-165.));
#6168=CARTESIAN_POINT('',(16.,46.,-165.));
#6169=CARTESIAN_POINT('',(-24.,-20.,-165.));
#6170=CARTESIAN_POINT('',(24.,-46.,-165.));
#6171=CARTESIAN_POINT('Origin',(0.,15.,-71.));
#6172=CARTESIAN_POINT('',(0.,15.,-71.));
#6173=CARTESIAN_POINT('',(44.,-29.,-71.));
#6174=CARTESIAN_POINT('',(44.,-29.,-71.));
#6175=CARTESIAN_POINT('',(44.,-21.,-71.));
#6176=CARTESIAN_POINT('',(44.,-29.,-71.));
#6177=CARTESIAN_POINT('',(44.,-21.,-71.));
#6178=CARTESIAN_POINT('',(44.,21.,-71.));
#6179=CARTESIAN_POINT('',(44.,21.,-71.));
#6180=CARTESIAN_POINT('',(44.,29.,-71.));
#6181=CARTESIAN_POINT('',(44.,29.,-71.));
#6182=CARTESIAN_POINT('',(44.,29.,-71.));
#6183=CARTESIAN_POINT('',(16.,48.,-71.));
#6184=CARTESIAN_POINT('',(24.,48.,-71.));
#6185=CARTESIAN_POINT('',(16.,-48.,-71.));
#6186=CARTESIAN_POINT('',(16.,48.,-71.));
#6187=CARTESIAN_POINT('',(24.,-48.,-71.));
#6188=CARTESIAN_POINT('Origin',(0.,31.5,6.12303176911193E-17));
#6189=CARTESIAN_POINT('',(0.,-31.5,6.12303176911193E-17));
#6190=CARTESIAN_POINT('Origin',(0.,0.,6.09863722023096E-17));
#6191=CARTESIAN_POINT('',(0.,31.5,6.12303176911193E-17));
#6192=CARTESIAN_POINT('Origin',(0.,0.,-14.));
#6193=CARTESIAN_POINT('',(0.,0.,176.4));
#6194=CARTESIAN_POINT('Origin',(0.,55.,-63.));
#6195=CARTESIAN_POINT('',(0.,55.,-63.));
#6196=CARTESIAN_POINT('Origin',(0.,22.,-63.));
#6197=CARTESIAN_POINT('',(0.,22.,-63.));
#6198=CARTESIAN_POINT('Origin',(0.,23.5,-46.));
#6199=CARTESIAN_POINT('',(0.,23.5,-46.));
#6200=CARTESIAN_POINT('Origin',(16.,-67.,-127.));
#6201=CARTESIAN_POINT('',(16.,-20.,-127.));
#6202=CARTESIAN_POINT('',(16.,-74.4030339164196,-133.7227292696));
#6203=CARTESIAN_POINT('',(16.,-74.4030339164196,-133.7227292696));
#6204=CARTESIAN_POINT('',(16.,-74.426181142428,-120.302848841496));
#6205=CARTESIAN_POINT('Origin',(16.,-67.,-127.));
#6206=CARTESIAN_POINT('',(16.,-48.,-91.));
#6207=CARTESIAN_POINT('',(16.,-48.,-91.));
#6208=CARTESIAN_POINT('',(16.,-48.,-71.));
#6209=CARTESIAN_POINT('',(16.,48.,-91.));
#6210=CARTESIAN_POINT('',(16.,48.,-71.));
#6211=CARTESIAN_POINT('',(16.,74.426181142428,-120.302848841496));
#6212=CARTESIAN_POINT('',(16.,48.,-91.));
#6213=CARTESIAN_POINT('',(16.,74.4030339164196,-133.7227292696));
#6214=CARTESIAN_POINT('Origin',(16.,67.,-127.));
#6215=CARTESIAN_POINT('',(16.,46.,-165.));
#6216=CARTESIAN_POINT('',(16.,74.4030339164196,-133.7227292696));
#6217=CARTESIAN_POINT('',(16.,20.,-165.));
#6218=CARTESIAN_POINT('',(16.,46.,-165.));
#6219=CARTESIAN_POINT('',(16.,20.,-127.));
#6220=CARTESIAN_POINT('',(16.,-67.,-153.));
#6221=CARTESIAN_POINT('Origin',(24.,-48.,-71.));
#6222=CARTESIAN_POINT('',(24.,-48.,-91.));
#6223=CARTESIAN_POINT('Origin',(24.,-48.,-91.));
#6224=CARTESIAN_POINT('',(24.,-74.426181142428,-120.302848841496));
#6225=CARTESIAN_POINT('Origin',(24.,-67.,-127.));
#6226=CARTESIAN_POINT('',(24.,-74.4030339164196,-133.7227292696));
#6227=CARTESIAN_POINT('Origin',(24.,-74.4030339164196,-133.7227292696));
#6228=CARTESIAN_POINT('Origin',(24.,46.,-165.));
#6229=CARTESIAN_POINT('',(-24.,20.,-165.));
#6230=CARTESIAN_POINT('',(24.,46.,-165.));
#6231=CARTESIAN_POINT('Origin',(24.,74.4030339164196,-133.7227292696));
#6232=CARTESIAN_POINT('',(24.,74.4030339164196,-133.7227292696));
#6233=CARTESIAN_POINT('Origin',(24.,67.,-127.));
#6234=CARTESIAN_POINT('',(24.,74.426181142428,-120.302848841496));
#6235=CARTESIAN_POINT('Origin',(24.,48.,-91.));
#6236=CARTESIAN_POINT('',(24.,48.,-91.));
#6237=CARTESIAN_POINT('Origin',(24.,48.,-71.));
#6238=CARTESIAN_POINT('Origin',(44.,29.,-71.));
#6239=CARTESIAN_POINT('',(44.,21.,-71.));
#6240=CARTESIAN_POINT('',(44.,29.,-71.));
#6241=CARTESIAN_POINT('Origin',(24.,29.,-71.));
#6242=CARTESIAN_POINT('Origin',(24.,21.,-71.));
#6243=CARTESIAN_POINT('Origin',(44.,-29.,-71.));
#6244=CARTESIAN_POINT('',(44.,-21.,-71.));
#6245=CARTESIAN_POINT('',(44.,-29.,-71.));
#6246=CARTESIAN_POINT('Origin',(24.,-29.,-71.));
#6247=CARTESIAN_POINT('Origin',(24.,-21.,-71.));
#6248=CARTESIAN_POINT('Origin',(-24.,-20.,-153.));
#6249=CARTESIAN_POINT('Origin',(-24.,20.,-153.));
#6250=CARTESIAN_POINT('Origin',(23.,-19.,-153.));
#6251=CARTESIAN_POINT('',(0.,19.,-153.));
#6252=CARTESIAN_POINT('',(23.,19.,-153.));
#6253=CARTESIAN_POINT('',(0.,-19.,-153.));
#6254=CARTESIAN_POINT('',(0.,-19.,-153.));
#6255=CARTESIAN_POINT('',(0.,-19.,-153.));
#6256=CARTESIAN_POINT('',(23.,-19.,-153.));
#6257=CARTESIAN_POINT('Origin',(23.,-19.,-165.));
#6258=CARTESIAN_POINT('',(0.,19.,-165.));
#6259=CARTESIAN_POINT('',(0.,-19.,-165.));
#6260=CARTESIAN_POINT('',(23.,19.,-165.));
#6261=CARTESIAN_POINT('',(23.,19.,-165.));
#6262=CARTESIAN_POINT('',(23.,-19.,-165.));
#6263=CARTESIAN_POINT('',(23.,19.,-165.));
#6264=CARTESIAN_POINT('',(0.,-19.,-165.));
#6265=CARTESIAN_POINT('',(23.,-19.,-165.));
#6266=CARTESIAN_POINT('',(0.,-19.,-165.));
#6267=CARTESIAN_POINT('Origin',(23.,19.,-165.));
#6268=CARTESIAN_POINT('',(23.,-19.,-165.));
#6269=CARTESIAN_POINT('',(23.,19.,-165.));
#6270=CARTESIAN_POINT('Origin',(23.,-19.,-165.));
#6271=CARTESIAN_POINT('',(0.,-19.,-165.));
#6272=CARTESIAN_POINT('Origin',(23.,19.,-165.));
#6273=CARTESIAN_POINT('',(0.,19.,-165.));
#6274=CARTESIAN_POINT('Origin',(0.,93.,313.849585789117));
#6275=CARTESIAN_POINT('Origin',(0.,93.,313.849585789117));
#6276=CARTESIAN_POINT('Origin',(0.,93.,313.849585789117));
#6277=CARTESIAN_POINT('Origin',(34.,-41.,-147.));
#6278=CARTESIAN_POINT('Origin',(34.,41.,-147.));
#7766=UNCERTAINTY_MEASURE_WITH_UNIT(LENGTH_MEASURE(0.01),#7784,
'DISTANCE_ACCURACY_VALUE',
'Maximum model space distance between geometric entities at asserted c
onnectivities');
#7773=UNCERTAINTY_MEASURE_WITH_UNIT(LENGTH_MEASURE(0.01),#7784,
'DISTANCE_ACCURACY_VALUE',
'Maximum model space distance between geometric entities at asserted c
onnectivities');
#7776=(
GEOMETRIC_REPRESENTATION_CONTEXT(3)
GLOBAL_UNCERTAINTY_ASSIGNED_CONTEXT((#7766))
GLOBAL_UNIT_ASSIGNED_CONTEXT((#7784,#7786,#7787))
REPRESENTATION_CONTEXT('','3D')
);
#7783=(
GEOMETRIC_REPRESENTATION_CONTEXT(3)
GLOBAL_UNCERTAINTY_ASSIGNED_CONTEXT((#7773))
GLOBAL_UNIT_ASSIGNED_CONTEXT((#7784,#7786,#7787))
REPRESENTATION_CONTEXT('','3D')
);
#7784=(
LENGTH_UNIT()
NAMED_UNIT(*)
SI_UNIT(.MILLI.,.METRE.)
);
#7786=(
NAMED_UNIT(*)
PLANE_ANGLE_UNIT()
SI_UNIT($,.RADIAN.)
);
#7787=(
NAMED_UNIT(*)
SI_UNIT($,.STERADIAN.)
SOLID_ANGLE_UNIT()
);
#7790=SHAPE_DEFINITION_REPRESENTATION(#7799,#7820);
#7799=PRODUCT_DEFINITION_SHAPE('',$,#7830);
#7820=SHAPE_REPRESENTATION('',(#4251),#7776);
#7827=PRODUCT_DEFINITION_CONTEXT('part definition',#7856,'design');
#7830=PRODUCT_DEFINITION('Body 1','Body 1',#7839,#7827);
#7839=PRODUCT_DEFINITION_FORMATION('',$,#7860);
#7856=APPLICATION_CONTEXT(
'Core Data for Automotive Mechanical Design Process');
#7857=PRODUCT_CONTEXT('part definition',#7856,'mechanical');
#7860=PRODUCT('Body 1','Body 1',$,(#7857));
#7868=PRESENTATION_STYLE_ASSIGNMENT((#7873));
#7873=SURFACE_STYLE_USAGE(.BOTH.,#7878);
#7878=SURFACE_SIDE_STYLE('',(#7883));
#7883=SURFACE_STYLE_FILL_AREA(#7888);
#7888=FILL_AREA_STYLE('Opaque(61,176,222)',(#7893));
#7893=FILL_AREA_STYLE_COLOUR('Opaque(61,176,222)',#7898);
#7898=COLOUR_RGB('Opaque(61,176,222)',0.23921568627451,0.690196078431373,
0.870588235294118);
ENDSEC;
END-ISO-10303-21;
